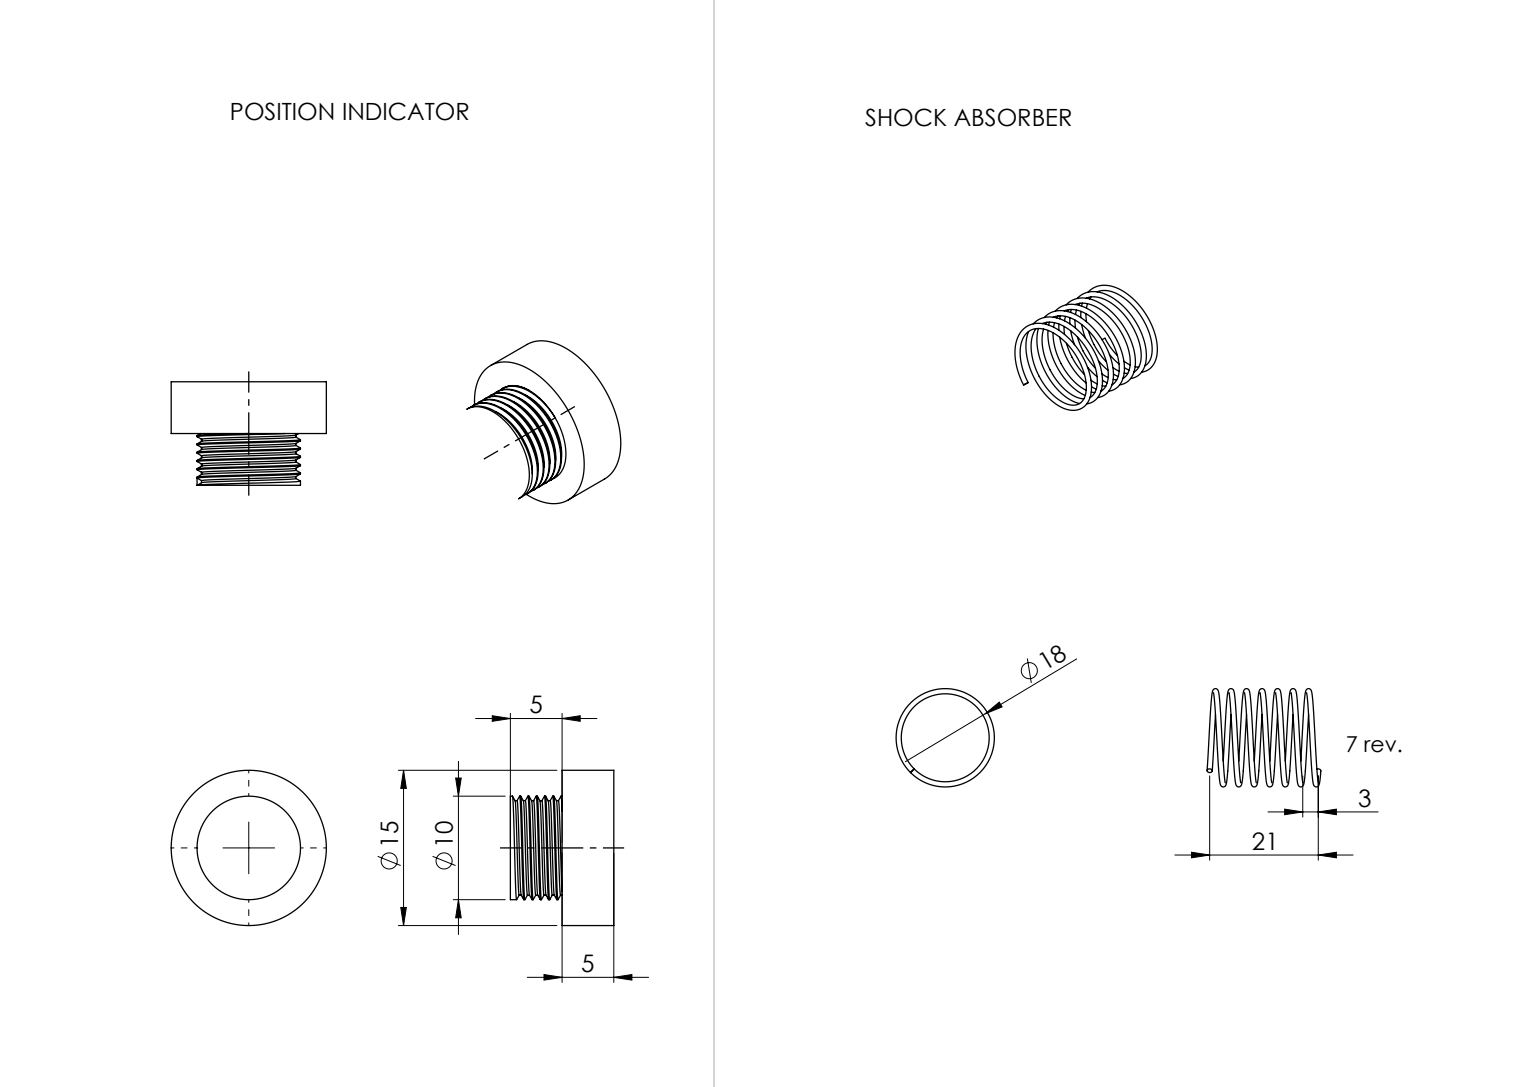
ISO-10303-21;
HEADER;
FILE_DESCRIPTION (('STEP AP214'),
    '1' );
FILE_NAME ('position indicator.step',
    '2026-09-29T11:11:29',
    ( '' ),
    ( '' ),
    'SwSTEP 2.0',
    'SolidWorks 2026',
    '' );
FILE_SCHEMA (( 'AUTOMOTIVE_DESIGN' ));
ENDSEC;

DATA;
#10=FACE_OUTER_BOUND ( 'NONE', #2337, .T. ) ;
#13=CARTESIAN_POINT ( 'NONE',  ( 5.000000000000000000, -47.07106781186545419, -99.34999999781506119 ) ) ;
#14=CARTESIAN_POINT ( 'NONE',  ( -4.566987299999997418, -46.89170807884566727, -96.79999999890753770 ) ) ;
#21=ORIENTED_EDGE ( 'NONE', *, *, #3963, .T. ) ;
#26=CARTESIAN_POINT ( 'NONE',  ( 5.000000000000000000, -47.07106781186545419, -98.54999999781504982 ) ) ;
#27=CARTESIAN_POINT ( 'NONE',  ( 3.535533905932737309, -48.53553390593270933, -96.29999999999999716 ) ) ;
#28=CARTESIAN_POINT ( 'NONE',  ( 9.184850993605145972E-16, -49.99999999999997158, -98.79999999999999716 ) ) ;
#29=ORIENTED_EDGE ( 'NONE', *, *, #4037, .T. ) ;
#33=EDGE_LOOP ( 'NONE', ( #4493, #8102, #3029, #2233, #7688, #6196, #940, #4526, #7806, #8045, #8010, #3978, #7053, #8494, #982 ) ) ;
#34=CARTESIAN_POINT ( 'NONE',  ( 3.229347689422839895, -41.77065231057713390, -98.94999999890752918 ) ) ;
#35=CARTESIAN_POINT ( 'NONE',  ( -4.999999999999997335, -47.07106781186546129, -97.24999999781506688 ) ) ;
#37=CARTESIAN_POINT ( 'NONE',  ( -3.229347689422840784, -41.77065231057713390, -98.54999999890752349 ) ) ;
#38=CARTESIAN_POINT ( 'NONE',  ( 0.000000000000000000, -44.99999999999997158, -100.0000000000000000 ) ) ;
#42=CARTESIAN_POINT ( 'NONE',  ( -3.535533905932735532, -48.53553390593270933, -98.09300000002185982 ) ) ;
#56=CARTESIAN_POINT ( 'NONE',  ( 4.999999999999998224, -42.92893218813449607, -99.24999999781505267 ) ) ;
#60=ADVANCED_FACE ( 'NONE', ( #2297 ), #6169, .T. ) ;
#68=CARTESIAN_POINT ( 'NONE',  ( 4.566987300000000083, -46.89170807884565306, -95.89999999890753202 ) ) ;
#71=VERTEX_POINT ( 'NONE', #7660 ) ;
#75=ORIENTED_EDGE ( 'NONE', *, *, #6394, .T. ) ;
#78=CARTESIAN_POINT ( 'NONE',  ( -1.891708078845683705, -49.56698729999997255, -97.69999999890751496 ) ) ;
#79=CARTESIAN_POINT ( 'NONE',  ( -3.535533905932736864, -41.46446609406723383, -95.79999999781504982 ) ) ;
#81=CARTESIAN_POINT ( 'NONE',  ( -4.566987299999997418, -46.89170807884566727, -99.99999999890754054 ) ) ;
#88=CARTESIAN_POINT ( 'NONE',  ( -4.999999999999998224, -42.92893218813448897, -96.64300000002185698 ) ) ;
#102=FACE_OUTER_BOUND ( 'NONE', #7927, .T. ) ;
#107=CARTESIAN_POINT ( 'NONE',  ( 9.184850993605145972E-16, -49.99999999999997158, -98.79999999999999716 ) ) ;
#114=CARTESIAN_POINT ( 'NONE',  ( 4.566987300000000083, -46.89170807884564596, -95.69999999890752918 ) ) ;
#116=CARTESIAN_POINT ( 'NONE',  ( 0.000000000000000000, -44.99999999999997158, -95.00000000000000000 ) ) ;
#117=CARTESIAN_POINT ( 'NONE',  ( 3.229347689422841228, -48.22934768942280925, -96.74999999890751212 ) ) ;
#119=FACE_OUTER_BOUND ( 'NONE', #8547, .T. ) ;
#126=CARTESIAN_POINT ( 'NONE',  ( 1.891708078845685481, -49.56698729999997255, -96.79999999890752349 ) ) ;
#127=CARTESIAN_POINT ( 'NONE',  ( -3.061616997868382155E-16, -39.99999999999997158, -100.6999999978150555 ) ) ;
#129=CARTESIAN_POINT ( 'NONE',  ( 4.566987299999998307, -44.99999999999997158, -98.04999999890752349 ) ) ;
#130=EDGE_CURVE ( 'NONE', #858, #6099, #1687, .T. ) ;
#132=CARTESIAN_POINT ( 'NONE',  ( -3.061616997868382155E-16, -39.99999999999997158, -98.39300000002185698 ) ) ;
#133=CARTESIAN_POINT ( 'NONE',  ( 4.566987300000000083, -46.89170807884565306, -95.69999999890755760 ) ) ;
#147=CARTESIAN_POINT ( 'NONE',  ( 1.308739421796400793, -40.13013661665839038, -99.99999999999998579 ) ) ;
#149=( NAMED_UNIT ( * ) PLANE_ANGLE_UNIT ( ) SI_UNIT ( $, .RADIAN. ) );
#160=CARTESIAN_POINT ( 'NONE',  ( 3.229347689422841228, -48.22934768942280925, -97.34999999890753486 ) ) ;
#163=CARTESIAN_POINT ( 'NONE',  ( -4.566987299999997418, -46.89170807884566727, -98.59999999890753486 ) ) ;
#172=CARTESIAN_POINT ( 'NONE',  ( -2.071067811865475505, -49.99999999999997158, -98.74999999781503845 ) ) ;
#173=CARTESIAN_POINT ( 'NONE',  ( -3.229347689422839451, -48.22934768942280925, -100.1499999989075178 ) ) ;
#174=CARTESIAN_POINT ( 'NONE',  ( 5.000000000000000000, -47.07106781186545419, -98.54999999781504982 ) ) ;
#175=CARTESIAN_POINT ( 'NONE',  ( 0.000000000000000000, -44.99999999999997158, -100.0000000000000000 ) ) ;
#176=CARTESIAN_POINT ( 'NONE',  ( 4.566987300000000083, -46.89170807884565306, -97.29999999890750928 ) ) ;
#179=CARTESIAN_POINT ( 'NONE',  ( 4.999999999999998224, -42.92893218813448897, -99.34300000002184561 ) ) ;
#180=CARTESIAN_POINT ( 'NONE',  ( -1.891708078845683039, -40.43301269999998482, -96.19999999890752918 ) ) ;
#189=CYLINDRICAL_SURFACE ( 'NONE', #1544, 4.999999999999998224 ) ;
#196=VERTEX_POINT ( 'NONE', #4485 ) ;
#200=EDGE_LOOP ( 'NONE', ( #2778, #541, #7748, #7443, #585 ) ) ;
#201=CARTESIAN_POINT ( 'NONE',  ( -4.566987299999998307, -43.10829192115428299, -96.09999999890753486 ) ) ;
#204=CARTESIAN_POINT ( 'NONE',  ( 4.566987299999998307, -44.99999999999997158, -99.04999999890752349 ) ) ;
#213=CARTESIAN_POINT ( 'NONE',  ( 4.999999999999998224, -44.99999999999997158, -98.60000000000000853 ) ) ;
#214=ADVANCED_FACE ( 'NONE', ( #3002 ), #7128, .T. ) ;
#215=CARTESIAN_POINT ( 'NONE',  ( -3.535533905932735532, -48.53553390593270933, -100.3999999978150441 ) ) ;
#217=CARTESIAN_POINT ( 'NONE',  ( -3.229347689422840784, -41.77065231057713390, -99.34999999890753486 ) ) ;
#221=CARTESIAN_POINT ( 'NONE',  ( 9.184850993605145972E-16, -49.99999999999997158, -99.59300000002184561 ) ) ;
#241=CARTESIAN_POINT ( 'NONE',  ( 4.566987299999998307, -44.99999999999997158, -95.64999999890753202 ) ) ;
#245=CARTESIAN_POINT ( 'NONE',  ( -3.229347689422840784, -41.77065231057713390, -96.34999999890752065 ) ) ;
#246=CARTESIAN_POINT ( 'NONE',  ( 4.999999999999998224, -44.99999999999997158, -95.40000000000000568 ) ) ;
#256=CARTESIAN_POINT ( 'NONE',  ( -3.535533905932736864, -41.46446609406723383, -100.5999999978150470 ) ) ;
#257=EDGE_CURVE ( 'NONE', #6677, #2955, #1349, .T. ) ;
#258=CARTESIAN_POINT ( 'NONE',  ( -4.999999999999998224, -44.99999999999997158, -98.09999999781504698 ) ) ;
#259=CARTESIAN_POINT ( 'NONE',  ( -3.229347689422839451, -48.22934768942280925, -98.34999999890753486 ) ) ;
#264=CARTESIAN_POINT ( 'NONE',  ( 3.535533905932736420, -41.46446609406723383, -95.29999999999999716 ) ) ;
#269=CARTESIAN_POINT ( 'NONE',  ( 4.999999999999998224, -42.92893218813449607, -100.0499999978150640 ) ) ;
#272=CARTESIAN_POINT ( 'NONE',  ( -1.891708078845683039, -40.43301269999998482, -95.59999999890753486 ) ) ;
#281=ADVANCED_FACE ( 'NONE', ( #6423 ), #7751, .T. ) ;
#286=CARTESIAN_POINT ( 'NONE',  ( 1.891708078845682595, -40.43301269999998482, -97.89999999890753202 ) ) ;
#289=CARTESIAN_POINT ( 'NONE',  ( 3.229347689422839895, -41.77065231057713390, -96.54999999890752349 ) ) ;
#291=CARTESIAN_POINT ( 'NONE',  ( -3.229347689422839451, -48.22934768942280925, -98.54999999890752349 ) ) ;
#296=( GEOMETRIC_REPRESENTATION_CONTEXT ( 3 ) GLOBAL_UNCERTAINTY_ASSIGNED_CONTEXT ( ( #1750 ) ) GLOBAL_UNIT_ASSIGNED_CONTEXT ( ( #6287, #2077, #6826 ) ) REPRESENTATION_CONTEXT ( 'NONE', 'WORKASPACE' ) );
#299=DIRECTION ( 'NONE',  ( -1.000000000000000000, 0.000000000000000000, 0.000000000000000000 ) ) ;
#301=CARTESIAN_POINT ( 'NONE',  ( 9.184850993605145972E-16, -49.99999999999997158, -100.2999999978150498 ) ) ;
#304=CARTESIAN_POINT ( 'NONE',  ( -3.229347689422840784, -41.77065231057713390, -100.1499999989075320 ) ) ;
#305=ORIENTED_EDGE ( 'NONE', *, *, #5462, .T. ) ;
#308=CARTESIAN_POINT ( 'NONE',  ( -4.999999999999998224, -45.95670858091268940, -94.97690301168722726 ) ) ;
#309=CARTESIAN_POINT ( 'NONE',  ( -1.891708078845683483, -49.56698729999997255, -95.89999999890753202 ) ) ;
#311=CARTESIAN_POINT ( 'NONE',  ( -2.071067811865475061, -39.99999999999997158, -96.64999999781504414 ) ) ;
#330=CARTESIAN_POINT ( 'NONE',  ( 3.229347689422841228, -48.22934768942280925, -99.94999999890752918 ) ) ;
#332=CARTESIAN_POINT ( 'NONE',  ( 1.891708078845682595, -40.43301269999998482, -95.69999999890751496 ) ) ;
#339=DIRECTION ( 'NONE',  ( -1.000000000000000000, 0.000000000000000000, 0.000000000000000000 ) ) ;
#341=CARTESIAN_POINT ( 'NONE',  ( -2.995331045737738095E-16, -40.10825317499996601, -100.0624999997268958 ) ) ;
#343=CARTESIAN_POINT ( 'NONE',  ( 2.071067811865474173, -39.99999999999997158, -96.85000000000002274 ) ) ;
#347=CARTESIAN_POINT ( 'NONE',  ( 3.535533905932736420, -41.46446609406723383, -97.69999999999998863 ) ) ;
#348=CARTESIAN_POINT ( 'NONE',  ( 4.999999999999998224, -42.92893218813448897, -96.84999999781504698 ) ) ;
#351=ADVANCED_FACE ( 'NONE', ( #3786 ), #5764, .T. ) ;
#354=CARTESIAN_POINT ( 'NONE',  ( -4.999999999999997335, -47.07106781186546129, -97.24999999781505267 ) ) ;
#355=CARTESIAN_POINT ( 'NONE',  ( -4.566987299999998307, -44.99999999999997158, -95.24999999890752633 ) ) ;
#364=ADVANCED_FACE ( 'NONE', ( #6505 ), #5809, .T. ) ;
#365=CARTESIAN_POINT ( 'NONE',  ( -4.566987299999998307, -43.10829192115428299, -99.29999999890752349 ) ) ;
#371=CARTESIAN_POINT ( 'NONE',  ( 4.566987299999998307, -44.99999999999997158, -98.24999999890751212 ) ) ;
#384=CARTESIAN_POINT ( 'NONE',  ( -2.071067811865475505, -49.99999999999996447, -95.64999999999999147 ) ) ;
#388=CARTESIAN_POINT ( 'NONE',  ( -2.071067811865475061, -39.99999999999997158, -96.75000000000001421 ) ) ;
#389=CARTESIAN_POINT ( 'NONE',  ( -4.999999999999998224, -44.99999999999997158, -97.29999999781504982 ) ) ;
#393=CARTESIAN_POINT ( 'NONE',  ( -4.999999999999998224, -42.92893218813449607, -98.25000000000000000 ) ) ;
#398=ORIENTED_EDGE ( 'NONE', *, *, #4779, .F. ) ;
#402=CARTESIAN_POINT ( 'NONE',  ( -4.999999999999998224, -44.99999999999997158, -95.79999999999999716 ) ) ;
#407=CARTESIAN_POINT ( 'NONE',  ( -4.566987299999998307, -44.99999999999997158, -96.24999999890751212 ) ) ;
#409=ORIENTED_EDGE ( 'NONE', *, *, #2203, .F. ) ;
#420=CARTESIAN_POINT ( 'NONE',  ( -2.071067811865475061, -39.99999999999997158, -95.15000000000000568 ) ) ;
#421=ORIENTED_EDGE ( 'NONE', *, *, #5864, .T. ) ;
#423=B_SPLINE_CURVE_WITH_KNOTS ( 'NONE', 3,
 ( #808, #6973, #5609, #147, #3632, #5471 ),
 .UNSPECIFIED., .F., .F.,
 ( 4, 2, 4 ),
 ( 0.1250000000000000000, 0.1875000000000000000, 0.2500000000000000000 ),
 .UNSPECIFIED. ) ;
#426=CARTESIAN_POINT ( 'NONE',  ( -3.061616997868382155E-16, -39.99999999999997158, -99.20000000000000284 ) ) ;
#427=CARTESIAN_POINT ( 'NONE',  ( 2.528021161412670192, -49.35149720828152908, -99.99914980755436034 ) ) ;
#434=CARTESIAN_POINT ( 'NONE',  ( 0.000000000000000000, -44.99999999999997158, -95.00000000000000000 ) ) ;
#442=CARTESIAN_POINT ( 'NONE',  ( 1.891708078845685481, -49.56698729999997255, -98.19999999890752918 ) ) ;
#449=CARTESIAN_POINT ( 'NONE',  ( 1.891708078845682595, -40.43301269999998482, -98.09999999890750644 ) ) ;
#462=CARTESIAN_POINT ( 'NONE',  ( -3.535533905932736864, -41.46446609406723383, -97.50000000000000000 ) ) ;
#468=CARTESIAN_POINT ( 'NONE',  ( -3.061616997868382155E-16, -39.99999999999997158, -97.60000000000000853 ) ) ;
#472=CARTESIAN_POINT ( 'NONE',  ( 4.999999999999998224, -44.99999999999997158, -96.89999999781505835 ) ) ;
#482=CARTESIAN_POINT ( 'NONE',  ( -3.229347689422840784, -41.77065231057713390, -99.34999999890753486 ) ) ;
#486=EDGE_CURVE ( 'NONE', #2955, #4083, #3727, .T. ) ;
#488=CARTESIAN_POINT ( 'NONE',  ( -4.566987299999998307, -44.99999999999997158, -96.04999999890752349 ) ) ;
#502=CARTESIAN_POINT ( 'NONE',  ( 4.999999999999998224, -44.99999999999997158, -97.00000000000000000 ) ) ;
#503=CARTESIAN_POINT ( 'NONE',  ( -3.535533905932736864, -41.46446609406723383, -99.90000000000000568 ) ) ;
#512=CARTESIAN_POINT ( 'NONE',  ( 2.071067811865474173, -39.99999999999997158, -97.64999999999999147 ) ) ;
#514=CARTESIAN_POINT ( 'NONE',  ( -4.961280561519337162, -44.31574741195442613, -99.99919817926395638 ) ) ;
#515=EDGE_CURVE ( 'NONE', #71, #2692, #2215, .T. ) ;
#528=CARTESIAN_POINT ( 'NONE',  ( 4.999999999999998224, -42.92893218813449607, -96.15000000000000568 ) ) ;
#535=CARTESIAN_POINT ( 'NONE',  ( 4.566987299999998307, -44.99999999999997158, -96.44999999890752918 ) ) ;
#541=ORIENTED_EDGE ( 'NONE', *, *, #2221, .F. ) ;
#547=CARTESIAN_POINT ( 'NONE',  ( 3.535533905932736420, -41.46446609406723383, -95.99999999781503845 ) ) ;
#553=CARTESIAN_POINT ( 'NONE',  ( -4.566987299999998307, -43.10829192115428299, -95.49999999890754054 ) ) ;
#554=CARTESIAN_POINT ( 'NONE',  ( 4.999999999999998224, -44.99999999999997158, -97.69999999781505551 ) ) ;
#557=CARTESIAN_POINT ( 'NONE',  ( -3.229347689422839451, -48.22934768942280925, -99.14999999890753202 ) ) ;
#558=CARTESIAN_POINT ( 'NONE',  ( -2.227513643315880643, -40.48620403085396902, -99.99969435636208459 ) ) ;
#561=CARTESIAN_POINT ( 'NONE',  ( 3.535533905932737309, -48.53553390593270933, -97.09300000002185982 ) ) ;
#564=( GEOMETRIC_REPRESENTATION_CONTEXT ( 3 ) GLOBAL_UNCERTAINTY_ASSIGNED_CONTEXT ( ( #7738 ) ) GLOBAL_UNIT_ASSIGNED_CONTEXT ( ( #896, #4163, #2803 ) ) REPRESENTATION_CONTEXT ( 'NONE', 'WORKASPACE' ) );
#578=CARTESIAN_POINT ( 'NONE',  ( 4.566987300000000083, -46.89170807884565306, -99.09999999890752065 ) ) ;
#581=CARTESIAN_POINT ( 'NONE',  ( -4.999999999999998224, -44.99999999999997158, -95.00000000000000000 ) ) ;
#585=ORIENTED_EDGE ( 'NONE', *, *, #701, .F. ) ;
#591=CARTESIAN_POINT ( 'NONE',  ( 4.999999999999998224, -44.99999999999997158, -98.49999999781503845 ) ) ;
#592=CARTESIAN_POINT ( 'NONE',  ( 3.535533905932737309, -48.53553390593270933, -98.59999999781504698 ) ) ;
#593=CARTESIAN_POINT ( 'NONE',  ( 4.999999999999998224, -44.99999999999997158, -95.00000000000000000 ) ) ;
#594=CARTESIAN_POINT ( 'NONE',  ( 3.535533905932736420, -41.46446609406723383, -99.29999999999999716 ) ) ;
#599=CARTESIAN_POINT ( 'NONE',  ( -3.229347689422840784, -41.77065231057713390, -98.74999999890751212 ) ) ;
#600=CARTESIAN_POINT ( 'NONE',  ( -4.999999999999998224, -45.95670858091268940, -95.67690300950226856 ) ) ;
#602=CARTESIAN_POINT ( 'NONE',  ( 4.566987300000000083, -46.89170807884565306, -97.29999999890750928 ) ) ;
#603=CARTESIAN_POINT ( 'NONE',  ( -4.111674810624561971, -47.85923343201969260, -99.99917207927896357 ) ) ;
#607=CARTESIAN_POINT ( 'NONE',  ( -2.071067811865475061, -39.99999999999997158, -97.54300000002184845 ) ) ;
#614=EDGE_LOOP ( 'NONE', ( #6274, #1845, #5331, #7137 ) ) ;
#619=ADVANCED_FACE ( 'NONE', ( #8516 ), #6422, .T. ) ;
#622=CARTESIAN_POINT ( 'NONE',  ( 4.999999999999998224, -44.99999999999997158, -99.29999999781504982 ) ) ;
#624=CARTESIAN_POINT ( 'NONE',  ( -4.566987299999997418, -46.89170807884566727, -99.39999999890751781 ) ) ;
#634=EDGE_LOOP ( 'NONE', ( #2546, #1880, #6420, #7835 ) ) ;
#639=CARTESIAN_POINT ( 'NONE',  ( 1.891708078845682595, -40.43301269999998482, -95.69999999890751496 ) ) ;
#640=CARTESIAN_POINT ( 'NONE',  ( -3.535533905932735532, -48.53553390593270933, -96.50000000000000000 ) ) ;
#641=CARTESIAN_POINT ( 'NONE',  ( -2.071067811865475061, -39.99999999999997158, -99.94999999999998863 ) ) ;
#647=CARTESIAN_POINT ( 'NONE',  ( -1.891708078845683705, -49.56698729999997255, -99.29999999890752349 ) ) ;
#648=CARTESIAN_POINT ( 'NONE',  ( 2.071067811865477282, -49.99999999999996447, -99.54999999999998295 ) ) ;
#650=CARTESIAN_POINT ( 'NONE',  ( 4.566987299999998307, -44.99999999999997158, -98.84999999890753486 ) ) ;
#656=CARTESIAN_POINT ( 'NONE',  ( 4.999999999999998224, -42.92893218813448897, -97.74300000002186550 ) ) ;
#666=ADVANCED_FACE ( 'NONE', ( #7216 ), #4530, .T. ) ;
#672=CARTESIAN_POINT ( 'NONE',  ( 8.389419568037416259E-16, -49.56698729999997255, -100.0499999989075093 ) ) ;
#681=ORIENTED_EDGE ( 'NONE', *, *, #1766, .F. ) ;
#685=CARTESIAN_POINT ( 'NONE',  ( -4.566987299999998307, -44.99999999999997158, -95.44999999890751496 ) ) ;
#687=CARTESIAN_POINT ( 'NONE',  ( 5.000000000000000000, -47.07106781186545419, -99.45000000000000284 ) ) ;
#688=ORIENTED_EDGE ( 'NONE', *, *, #7144, .T. ) ;
#692=ORIENTED_EDGE ( 'NONE', *, *, #3230, .T. ) ;
#693=CARTESIAN_POINT ( 'NONE',  ( 4.566987300000000083, -46.89170807884564596, -97.49999999890752633 ) ) ;
#694=CARTESIAN_POINT ( 'NONE',  ( 4.999999999999998224, -42.92893218813448897, -99.35000000000000853 ) ) ;
#696=CARTESIAN_POINT ( 'NONE',  ( -2.796473189345805913E-16, -40.43301269999997061, -97.04999999890752349 ) ) ;
#700=CARTESIAN_POINT ( 'NONE',  ( -3.061616997868382155E-16, -39.99999999999997158, -95.99300000002185129 ) ) ;
#701=EDGE_CURVE ( 'NONE', #2848, #7832, #7939, .T. ) ;
#707=ORIENTED_EDGE ( 'NONE', *, *, #8464, .T. ) ;
#723=EDGE_CURVE ( 'NONE', #4083, #876, #2542, .T. ) ;
#729=CARTESIAN_POINT ( 'NONE',  ( -4.999999999999998224, -44.99999999999997158, -100.4999999978150385 ) ) ;
#732=( BOUNDED_CURVE ( )  B_SPLINE_CURVE ( 2, ( #402, #3161, #7865, #3114, #1829, #4510, #7198, #528, #4072 ),
 .UNSPECIFIED., .F., .T. ) 
 B_SPLINE_CURVE_WITH_KNOTS ( ( 3, 2, 2, 2, 3 ),
 ( 0.1428571428571428215, 0.1607142857142856984, 0.1785714285714285476, 0.1964285714285714246, 0.2142857142857142738 ),
 .UNSPECIFIED. ) 
 CURVE ( )  GEOMETRIC_REPRESENTATION_ITEM ( )  RATIONAL_B_SPLINE_CURVE ( ( 1.000000000000000222, 0.9238795325112866275, 1.000000000000000000, 0.9238795325112867385, 1.000000000000000000, 0.9238795325112867385, 1.000000000000000000, 0.9238795325112867385, 1.000000000000000000 ) ) 
 REPRESENTATION_ITEM ( '' )  );
#740=CARTESIAN_POINT ( 'NONE',  ( -4.566987299999998307, -44.99999999999997158, -97.84999999890752065 ) ) ;
#741=CARTESIAN_POINT ( 'NONE',  ( 3.535533905932737309, -48.53553390593270933, -99.50000000000000000 ) ) ;
#743=CARTESIAN_POINT ( 'NONE',  ( 3.229347689422841228, -48.22934768942280925, -97.34999999890753486 ) ) ;
#744=SURFACE_SIDE_STYLE ('',( #4672 ) ) ;
#747=CARTESIAN_POINT ( 'NONE',  ( -4.999999999999998224, -42.92893218813448897, -95.04300000002184845 ) ) ;
#753=ORIENTED_EDGE ( 'NONE', *, *, #7226, .F. ) ;
#758=DIRECTION ( 'NONE',  ( 0.000000000000000000, 0.000000000000000000, 1.000000000000000000 ) ) ;
#765=CARTESIAN_POINT ( 'NONE',  ( 4.999999999999998224, -44.99999999999997158, -98.60000000000000853 ) ) ;
#773=CARTESIAN_POINT ( 'NONE',  ( -4.566987299999998307, -44.99999999999997158, -100.0499999989075235 ) ) ;
#775=CARTESIAN_POINT ( 'NONE',  ( -2.071067811865475505, -49.99999999999996447, -98.74999999781503845 ) ) ;
#782=AXIS2_PLACEMENT_3D ( 'NONE', #1939, #5036, #8351 ) ;
#785=CARTESIAN_POINT ( 'NONE',  ( -1.891708078845683705, -49.56698729999997255, -98.49999999890752633 ) ) ;
#786=EDGE_CURVE ( 'NONE', #5319, #2418, #5107, .T. ) ;
#787=CARTESIAN_POINT ( 'NONE',  ( 4.999999999999998224, -42.92893218813448897, -100.0499999978150356 ) ) ;
#789=CARTESIAN_POINT ( 'NONE',  ( 3.229347689422841228, -48.22934768942280925, -98.14999999890753202 ) ) ;
#790=PLANE ( 'NONE',  #5639 ) ;
#793=EDGE_CURVE ( 'NONE', #5525, #6251, #3781, .T. ) ;
#794=CARTESIAN_POINT ( 'NONE',  ( 3.535533905932736420, -41.46446609406723383, -99.29300000002184845 ) ) ;
#797=FACE_OUTER_BOUND ( 'NONE', #8191, .T. ) ;
#799=VERTEX_POINT ( 'NONE', #8543 ) ;
#800=CARTESIAN_POINT ( 'NONE',  ( 4.999999999999998224, -44.99999999999997158, -100.0999999978150470 ) ) ;
#808=CARTESIAN_POINT ( 'NONE',  ( 3.535533969928884801, -41.46446615806338087, -100.0000000000000142 ) ) ;
#811=CARTESIAN_POINT ( 'NONE',  ( 2.071067811865477282, -49.99999999999997158, -98.75000000000001421 ) ) ;
#816=ORIENTED_EDGE ( 'NONE', *, *, #1726, .T. ) ;
#817=CARTESIAN_POINT ( 'NONE',  ( 4.566987299999998307, -43.10829192115428299, -97.19999999890751496 ) ) ;
#821=CARTESIAN_POINT ( 'NONE',  ( 3.229347689422839895, -41.77065231057713390, -97.34999999890752065 ) ) ;
#832=CARTESIAN_POINT ( 'NONE',  ( 3.229347689422841228, -48.22934768942280925, -98.94999999890752918 ) ) ;
#835=CARTESIAN_POINT ( 'NONE',  ( -2.071067811865475061, -39.99999999999997158, -95.15000000000000568 ) ) ;
#836=CARTESIAN_POINT ( 'NONE',  ( 4.566987299999998307, -44.99999999999997158, -96.44999999890752918 ) ) ;
#838=AXIS2_PLACEMENT_3D ( 'NONE', #8397, #5741, #2402 ) ;
#858=VERTEX_POINT ( 'NONE', #591 ) ;
#861=CARTESIAN_POINT ( 'NONE',  ( -2.796473189345805913E-16, -40.43301269999997061, -98.04999999890752349 ) ) ;
#872=CARTESIAN_POINT ( 'NONE',  ( -3.229347689422840784, -41.77065231057713390, -100.3499999989075206 ) ) ;
#873=CARTESIAN_POINT ( 'NONE',  ( -4.999999999999998224, -42.92893218813448897, -98.94999999781504130 ) ) ;
#875=CARTESIAN_POINT ( 'NONE',  ( -1.891708078845683483, -49.56698729999997255, -97.49999999890754054 ) ) ;
#876=VERTEX_POINT ( 'NONE', #8711 ) ;
#879=CARTESIAN_POINT ( 'NONE',  ( -4.999999999999997335, -47.07106781186546129, -98.14300000002184277 ) ) ;
#891=CARTESIAN_POINT ( 'NONE',  ( 0.000000000000000000, -44.99999999999997158, -95.00000000000000000 ) ) ;
#896=( LENGTH_UNIT ( ) NAMED_UNIT ( * ) SI_UNIT ( .MILLI., .METRE. ) );
#905=CARTESIAN_POINT ( 'NONE',  ( -1.891708078845683039, -40.43301269999998482, -100.1999999989075150 ) ) ;
#908=CARTESIAN_POINT ( 'NONE',  ( -3.229347689422840784, -41.77065231057713390, -97.14999999890753202 ) ) ;
#910=CARTESIAN_POINT ( 'NONE',  ( 4.999999999999998224, -44.99999999999997158, -96.09999999781504698 ) ) ;
#916=EDGE_CURVE ( 'NONE', #5583, #5143, #1973, .T. ) ;
#918=CARTESIAN_POINT ( 'NONE',  ( -3.535533905932735532, -48.53553390593270933, -98.79999999781504982 ) ) ;
#920=CARTESIAN_POINT ( 'NONE',  ( -4.999999999999998224, -44.99999999999997158, -98.09999999781504698 ) ) ;
#921=CARTESIAN_POINT ( 'NONE',  ( 9.184850993605145972E-16, -49.99999999999997158, -97.89999999781504414 ) ) ;
#922=CARTESIAN_POINT ( 'NONE',  ( -1.891708078845683483, -49.56698729999997255, -99.89999999890753202 ) ) ;
#927=CARTESIAN_POINT ( 'NONE',  ( -3.535533905932736864, -41.46446609406723383, -99.89300000002185698 ) ) ;
#928=CARTESIAN_POINT ( 'NONE',  ( 4.566987299999998307, -43.10829192115428299, -95.59999999890754907 ) ) ;
#930=CARTESIAN_POINT ( 'NONE',  ( 5.000000000000000000, -47.07106781186545419, -96.94999999781504130 ) ) ;
#940=ORIENTED_EDGE ( 'NONE', *, *, #4323, .F. ) ;
#948=CARTESIAN_POINT ( 'NONE',  ( -2.796473189345805913E-16, -40.43301269999997061, -97.84999999890753486 ) ) ;
#951=CARTESIAN_POINT ( 'NONE',  ( -3.229347689422839451, -48.22934768942280925, -97.74999999890751212 ) ) ;
#953=CARTESIAN_POINT ( 'NONE',  ( 4.566987299999998307, -43.10829192115428299, -96.59999999890753486 ) ) ;
#954=LINE ( 'NONE', #2655, #1137 ) ;
#963=CARTESIAN_POINT ( 'NONE',  ( -4.999999999999998224, -44.99999999999997158, -99.69999999781505551 ) ) ;
#965=CARTESIAN_POINT ( 'NONE',  ( 4.566987299999998307, -44.99999999999997158, -98.84999999890753486 ) ) ;
#970=CARTESIAN_POINT ( 'NONE',  ( -3.535533905932736864, -41.46446609406723383, -98.29300000002184845 ) ) ;
#972=CARTESIAN_POINT ( 'NONE',  ( 4.999999999999998224, -44.99999999999997158, -97.69999999781505551 ) ) ;
#982=ORIENTED_EDGE ( 'NONE', *, *, #7961, .F. ) ;
#987=CARTESIAN_POINT ( 'NONE',  ( -1.891708078845683705, -49.56698729999997255, -99.09999999890753486 ) ) ;
#993=CARTESIAN_POINT ( 'NONE',  ( -4.566987299999998307, -43.10829192115428299, -97.89999999890751781 ) ) ;
#1002=LINE ( 'NONE', #8423, #4723 ) ;
#1003=DIRECTION ( 'NONE',  ( -1.000000000000000000, -6.123233995736960786E-17, 0.000000000000000000 ) ) ;
#1006=CARTESIAN_POINT ( 'NONE',  ( 9.184850993605145972E-16, -49.99999999999997158, -95.60000000000000853 ) ) ;
#1011=CARTESIAN_POINT ( 'NONE',  ( 4.999999999999998224, -44.99999999999997158, -99.40000000000000568 ) ) ;
#1013=CARTESIAN_POINT ( 'NONE',  ( 8.389419568037416259E-16, -49.56698729999997255, -95.84999999890753486 ) ) ;
#1015=CARTESIAN_POINT ( 'NONE',  ( 3.535533905932736420, -41.46446609406723383, -97.59999999781504698 ) ) ;
#1023=CARTESIAN_POINT ( 'NONE',  ( 4.566987300000000083, -46.89170807884564596, -95.89999999890753202 ) ) ;
#1031=EDGE_LOOP ( 'NONE', ( #6594, #5096, #4196, #1185 ) ) ;
#1035=CARTESIAN_POINT ( 'NONE',  ( -4.999999999999998224, -44.99999999999997158, -95.00000000000000000 ) ) ;
#1040=CARTESIAN_POINT ( 'NONE',  ( 3.229347689422839895, -41.77065231057713390, -97.34999999890752065 ) ) ;
#1048=CARTESIAN_POINT ( 'NONE',  ( 0.000000000000000000, -44.99999999999997158, -95.00000000000000000 ) ) ;
#1050=CARTESIAN_POINT ( 'NONE',  ( -3.061616997868382155E-16, -39.99999999999997158, -97.49999999781503845 ) ) ;
#1052=CARTESIAN_POINT ( 'NONE',  ( 2.071067811865474173, -39.99999999999997158, -96.04999999999999716 ) ) ;
#1056=VERTEX_POINT ( 'NONE', #2815 ) ;
#1057=CARTESIAN_POINT ( 'NONE',  ( 9.184850993605145972E-16, -49.99999999999997158, -98.79999999999999716 ) ) ;
#1058=CARTESIAN_POINT ( 'NONE',  ( -3.535533905932735532, -48.53553390593270933, -97.99999999781503845 ) ) ;
#1066=( BOUNDED_SURFACE ( )  B_SPLINE_SURFACE ( 1, 2, ( 
 ( #1706, #4394, #3038, #1615, #4476, #332, #3648, #7162, #3816, #7083, #7743, #2333, #7120, #6326, #5841, #6455, #407, #4305, #2417, #5095, #1661, #2992, #5713, #953, #5137, #7700, #5669, #8371, #6371, #1755, #6497, #7829, #4352, #1082, #7786, #1122, #3079, #5013, #1040, #4437, #5798, #8531, #5053, #8414, #3120, #2378, #3776, #1794, #7032, #993, #3733, #8492, #2456, #449, #6414, #3691, #371, #4969, #5755, #6989, #3167, #7652, #291, #7955, #5927, #5888, #6052, #6621, #4606, #4563, #1333, #1918, #1247, #578, #8619, #3204, #7204, #4034, #8661, #624, #7913, #3945, #1959, #8574, #6712, #2587, #8700, #3903, #7871, #2538, #4646, #6010, #672, #7290, #2627, #8002, #1288, #5257, #5217, #3294, #2498 ),
 ( #5968, #5297, #1166, #3989, #7334, #3333, #6669, #4517, #1879, #3860, #2672, #5178, #5340, #7246, #8043, #2004, #488, #4696, #7381, #1207, #3378, #6580, #1835, #6539, #535, #3245, #2714, #2050, #4739, #5384, #8093, #14, #8681, #1358, #7359, #1313, #696, #6778, #2697, #6645, #6079, #602, #743, #5323, #3316, #5238, #4813, #7447, #4671, #7933, #5365, #4013, #1405, #3402, #8642, #4059, #3448, #4584, #8023, #8068, #1229, #6692, #2608, #5276, #2031, #1984, #37, #7980, #8596, #1942, #2740, #4719, #650, #3359, #8118, #4764, #7268, #5409, #557, #2561, #1900, #3268, #4627, #7311, #6737, #2076, #4101, #7403, #5948, #3926, #1268, #6601, #3968, #6034, #5990, #2654, #773, #8279, #7517, #905, #2241 ) ),
 .UNSPECIFIED., .F., .F., .T. ) 
 B_SPLINE_SURFACE_WITH_KNOTS ( ( 2, 2 ),
 ( 3, 2, 2, 2, 2, 2, 2, 2, 2, 2, 2, 2, 2, 2, 2, 2, 2, 2, 2, 2, 2, 2, 2, 2, 2, 2, 2, 2, 2, 2, 2, 2, 2, 2, 2, 2, 2, 2, 2, 2, 2, 2, 2, 2, 2, 2, 2, 2, 2, 2, 3 ),
 ( 0.000000000000000000, 1.000000000000000000 ),
 ( 0.000000000000000000, 0.01785714285714285615, 0.03571428571428571230, 0.05357142857142856845, 0.07142857142857142461, 0.08928571428571428770, 0.1071428571428571369, 0.1250000000000000000, 0.1428571428571428492, 0.1607142857142857262, 0.1785714285714285754, 0.1964285714285714246, 0.2142857142857142738, 0.2321428571428571508, 0.2500000000000000000, 0.2678571428571428492, 0.2857142857142856984, 0.3035714285714285476, 0.3214285714285714524, 0.3392857142857143016, 0.3571428571428571508, 0.3750000000000000000, 0.3928571428571428492, 0.4107142857142856984, 0.4285714285714285476, 0.4464285714285714524, 0.4642857142857143016, 0.4821428571428571508, 0.5000000000000000000, 0.5178571428571429047, 0.5357142857142856984, 0.5535714285714286031, 0.5714285714285713969, 0.5892857142857143016, 0.6071428571428570953, 0.6250000000000000000, 0.6428571428571429047, 0.6607142857142856984, 0.6785714285714286031, 0.6964285714285713969, 0.7142857142857143016, 0.7321428571428570953, 0.7500000000000000000, 0.7678571428571429047, 0.7857142857142856984, 0.8035714285714286031, 0.8214285714285713969, 0.8392857142857143016, 0.8571428571428570953, 0.8750000000000000000, 0.8928571428571429047 ),
 .UNSPECIFIED. ) 
 GEOMETRIC_REPRESENTATION_ITEM ( )  RATIONAL_B_SPLINE_SURFACE ( (
 ( 1.000000000000000000, 0.9238795325112867385, 1.000000000000000000, 0.9238795325112867385, 1.000000000000000000, 0.9238795325112867385, 1.000000000000000000, 0.9238795325112867385, 1.000000000000000000, 0.9238795325112867385, 1.000000000000000000, 0.9238795325112867385, 1.000000000000000000, 0.9238795325112867385, 1.000000000000000000, 0.9238795325112867385, 1.000000000000000000, 0.9238795325112867385, 1.000000000000000000, 0.9238795325112867385, 1.000000000000000000, 0.9238795325112867385, 1.000000000000000000, 0.9238795325112867385, 1.000000000000000000, 0.9238795325112867385, 1.000000000000000000, 0.9238795325112867385, 1.000000000000000000, 0.9238795325112867385, 1.000000000000000000, 0.9238795325112867385, 1.000000000000000000, 0.9238795325112867385, 1.000000000000000000, 0.9238795325112867385, 1.000000000000000000, 0.9238795325112867385, 1.000000000000000000, 0.9238795325112867385, 1.000000000000000000, 0.9238795325112867385, 1.000000000000000000, 0.9238795325112867385, 1.000000000000000000, 0.9238795325112867385, 1.000000000000000000, 0.9238795325112867385, 1.000000000000000000, 0.9238795325112867385, 1.000000000000000000, 0.9238795325112867385, 1.000000000000000000, 0.9238795325112867385, 1.000000000000000000, 0.9238795325112867385, 1.000000000000000000, 0.9238795325112867385, 1.000000000000000000, 0.9238795325112867385, 1.000000000000000000, 0.9238795325112867385, 1.000000000000000000, 0.9238795325112867385, 1.000000000000000000, 0.9238795325112867385, 1.000000000000000000, 0.9238795325112867385, 1.000000000000000000, 0.9238795325112867385, 1.000000000000000000, 0.9238795325112867385, 1.000000000000000000, 0.9238795325112867385, 1.000000000000000000, 0.9238795325112867385, 1.000000000000000000, 0.9238795325112867385, 1.000000000000000000, 0.9238795325112867385, 1.000000000000000000, 0.9238795325112867385, 1.000000000000000000, 0.9238795325112867385, 1.000000000000000000, 0.9238795325112867385, 1.000000000000000000, 0.9238795325112867385, 1.000000000000000000, 0.9238795325112867385, 1.000000000000000000, 0.9238795325112867385, 1.000000000000000000, 0.9238795325112867385, 1.000000000000000000, 0.9238795325112867385, 1.000000000000000000, 0.9238795325112867385, 1.000000000000000000, 0.9238795325112867385, 1.000000000000000000),
 ( 1.000000000000000000, 0.9238795325112867385, 1.000000000000000000, 0.9238795325112867385, 1.000000000000000000, 0.9238795325112867385, 1.000000000000000000, 0.9238795325112867385, 1.000000000000000000, 0.9238795325112867385, 1.000000000000000000, 0.9238795325112867385, 1.000000000000000000, 0.9238795325112867385, 1.000000000000000000, 0.9238795325112867385, 1.000000000000000000, 0.9238795325112867385, 1.000000000000000000, 0.9238795325112867385, 1.000000000000000000, 0.9238795325112867385, 1.000000000000000000, 0.9238795325112867385, 1.000000000000000000, 0.9238795325112867385, 1.000000000000000000, 0.9238795325112867385, 1.000000000000000000, 0.9238795325112867385, 1.000000000000000000, 0.9238795325112867385, 1.000000000000000000, 0.9238795325112867385, 1.000000000000000000, 0.9238795325112867385, 1.000000000000000000, 0.9238795325112867385, 1.000000000000000000, 0.9238795325112867385, 1.000000000000000000, 0.9238795325112867385, 1.000000000000000000, 0.9238795325112867385, 1.000000000000000000, 0.9238795325112867385, 1.000000000000000000, 0.9238795325112867385, 1.000000000000000000, 0.9238795325112867385, 1.000000000000000000, 0.9238795325112867385, 1.000000000000000000, 0.9238795325112867385, 1.000000000000000000, 0.9238795325112867385, 1.000000000000000000, 0.9238795325112867385, 1.000000000000000000, 0.9238795325112867385, 1.000000000000000000, 0.9238795325112867385, 1.000000000000000000, 0.9238795325112867385, 1.000000000000000000, 0.9238795325112867385, 1.000000000000000000, 0.9238795325112867385, 1.000000000000000000, 0.9238795325112867385, 1.000000000000000000, 0.9238795325112867385, 1.000000000000000000, 0.9238795325112867385, 1.000000000000000000, 0.9238795325112867385, 1.000000000000000000, 0.9238795325112867385, 1.000000000000000000, 0.9238795325112867385, 1.000000000000000000, 0.9238795325112867385, 1.000000000000000000, 0.9238795325112867385, 1.000000000000000000, 0.9238795325112867385, 1.000000000000000000, 0.9238795325112867385, 1.000000000000000000, 0.9238795325112867385, 1.000000000000000000, 0.9238795325112867385, 1.000000000000000000, 0.9238795325112867385, 1.000000000000000000, 0.9238795325112867385, 1.000000000000000000, 0.9238795325112867385, 1.000000000000000000, 0.9238795325112867385, 1.000000000000000000) ) ) 
 REPRESENTATION_ITEM ( '' )  SURFACE ( )  );
#1077=CARTESIAN_POINT ( 'NONE',  ( 8.389419568037416259E-16, -49.56698729999997255, -99.04999999890752349 ) ) ;
#1082=CARTESIAN_POINT ( 'NONE',  ( -4.566987299999998307, -43.10829192115428299, -97.09999999890752065 ) ) ;
#1093=CARTESIAN_POINT ( 'NONE',  ( -4.999999999999998224, -44.99999999999997158, -95.79999999999999716 ) ) ;
#1096=CARTESIAN_POINT ( 'NONE',  ( 4.999999999999998224, -44.99999999999997158, -95.40000000000000568 ) ) ;
#1101=CARTESIAN_POINT ( 'NONE',  ( -3.535533905932736864, -41.46446609406723383, -99.10000000000000853 ) ) ;
#1103=CARTESIAN_POINT ( 'NONE',  ( 4.270369862968768082, -42.33539640546668892, -99.99920780850642643 ) ) ;
#1105=ADVANCED_FACE ( 'NONE', ( #6898 ), #6943, .T. ) ;
#1116=CARTESIAN_POINT ( 'NONE',  ( -1.891708078845683039, -40.43301269999998482, -100.1999999989075292 ) ) ;
#1122=CARTESIAN_POINT ( 'NONE',  ( -1.891708078845683039, -40.43301269999998482, -97.19999999890752918 ) ) ;
#1133=CARTESIAN_POINT ( 'NONE',  ( -4.999999999999998224, -44.99999999999997158, -97.40000000000000568 ) ) ;
#1135=CARTESIAN_POINT ( 'NONE',  ( 2.071067811865477282, -49.99999999999996447, -97.15000000000000568 ) ) ;
#1137=VECTOR ( 'NONE', #1455, 1000.000000000000000 ) ;
#1141=CARTESIAN_POINT ( 'NONE',  ( 4.999999999999998224, -42.92893218813448897, -98.54999999999999716 ) ) ;
#1158=CARTESIAN_POINT ( 'NONE',  ( -4.566987299999997418, -46.89170807884566017, -98.39999999890753202 ) ) ;
#1160=AXIS2_PLACEMENT_3D ( 'NONE', #8260, #1369, #7455 ) ;
#1163=DIRECTION ( 'NONE',  ( -0.000000000000000000, -0.000000000000000000, 1.000000000000000000 ) ) ;
#1166=CARTESIAN_POINT ( 'NONE',  ( -3.229347689422840784, -41.77065231057713390, -95.34999999890753486 ) ) ;
#1180=CARTESIAN_POINT ( 'NONE',  ( -4.999999999999994671, -47.07106781186546840, -96.55000000000001137 ) ) ;
#1181=CARTESIAN_POINT ( 'NONE',  ( -2.071067811865475505, -49.99999999999996447, -98.85000000000002274 ) ) ;
#1185=ORIENTED_EDGE ( 'NONE', *, *, #2970, .F. ) ;
#1186=CARTESIAN_POINT ( 'NONE',  ( -4.999999999999998224, -44.99999999999997158, -97.40000000000000568 ) ) ;
#1207=CARTESIAN_POINT ( 'NONE',  ( -1.891708078845683039, -40.43301269999998482, -96.19999999890752918 ) ) ;
#1220=CARTESIAN_POINT ( 'NONE',  ( -4.999999999999998224, -44.99999999999997158, -99.79999999999999716 ) ) ;
#1221=ORIENTED_EDGE ( 'NONE', *, *, #5114, .F. ) ;
#1227=CARTESIAN_POINT ( 'NONE',  ( 5.000000000000000000, -47.07106781186545419, -96.25000000000000000 ) ) ;
#1229=CARTESIAN_POINT ( 'NONE',  ( 8.389419568037416259E-16, -49.56698729999997255, -98.24999999890752633 ) ) ;
#1233=CARTESIAN_POINT ( 'NONE',  ( 2.071067811865477282, -49.99999999999996447, -96.34300000002185982 ) ) ;
#1247=CARTESIAN_POINT ( 'NONE',  ( 4.566987299999998307, -44.99999999999997158, -99.04999999890752349 ) ) ;
#1250=LINE ( 'NONE', #3948, #2876 ) ;
#1258=CARTESIAN_POINT ( 'NONE',  ( 4.999999999999998224, -42.92893218813448897, -98.44999999781505551 ) ) ;
#1259=CARTESIAN_POINT ( 'NONE',  ( -3.535533905932735532, -48.53553390593270933, -98.10000000000000853 ) ) ;
#1264=CARTESIAN_POINT ( 'NONE',  ( 3.229347689422839895, -41.77065231057713390, -97.34999999890752065 ) ) ;
#1266=CARTESIAN_POINT ( 'NONE',  ( -2.071067811865475061, -39.99999999999997158, -99.94999999999998863 ) ) ;
#1268=CARTESIAN_POINT ( 'NONE',  ( 3.229347689422841228, -48.22934768942280925, -99.74999999890752633 ) ) ;
#1269=CARTESIAN_POINT ( 'NONE',  ( 4.766825771567327230, -43.38335435358479941, -100.0003056439282147 ) ) ;
#1272=CARTESIAN_POINT ( 'NONE',  ( -2.071067811865475505, -49.99999999999996447, -96.44300000002185413 ) ) ;
#1282=AXIS2_PLACEMENT_3D ( 'NONE', #1511, #4204, #6885 ) ;
#1283=CARTESIAN_POINT ( 'NONE',  ( -5.000000000000003553, -42.92893218813449607, -96.64999999999999147 ) ) ;
#1284=DIRECTION ( 'NONE',  ( -0.000000000000000000, -0.000000000000000000, -1.000000000000000000 ) ) ;
#1288=CARTESIAN_POINT ( 'NONE',  ( -4.566987299999998307, -44.99999999999997158, -100.2499999989075121 ) ) ;
#1289=AXIS2_PLACEMENT_3D ( 'NONE', #4498, #7851, #1977 ) ;
#1293=( BOUNDED_CURVE ( )  B_SPLINE_CURVE ( 2, ( #2605, #553, #3265, #272, #8396, #7061, #3021, #2974, #2316, #1023, #4994, #7727, #3715, #7678, #2358, #1641, #6734, #2028, #2121, #7444, #3444, #7356, #4716, #6219, #4098, #7486, #2073, #126, #1402, #3488, #2651, #7400, #4760, #6121, #4143, #4803, #2735, #2825, #1264, #5406, #6775, #693, #8020, #3399, #8064, #78, #4852, #2784, #740, #1355, #2693, #1451, #5449, #8115, #5497, #6689, #8207, #4054, #2166, #8161, #6822, #785, #3965, #6170, #3356, #6642, #599, #6076, #3313, #5987, #34, #8678, #5320, #1980, #4667, #1310, #4010, #647, #6031, #5362, #4184, #6208, #7661, #5586, #6866, #6910, #3003, #4894, #5721, #4227, #2340, #8293, #8250, #6954, #173, #2872, #5544, #8332, #872, #5021, #2209 ),
 .UNSPECIFIED., .F., .T. ) 
 B_SPLINE_CURVE_WITH_KNOTS ( ( 3, 2, 2, 2, 2, 2, 2, 2, 2, 2, 2, 2, 2, 2, 2, 2, 2, 2, 2, 2, 2, 2, 2, 2, 2, 2, 2, 2, 2, 2, 2, 2, 2, 2, 2, 2, 2, 2, 2, 2, 2, 2, 2, 2, 2, 2, 2, 2, 2, 2, 3 ),
 ( 0.000000000000000000, 0.01785714285714285615, 0.03571428571428571230, 0.05357142857142856845, 0.07142857142857142461, 0.08928571428571428770, 0.1071428571428571369, 0.1250000000000000000, 0.1428571428571428492, 0.1607142857142857262, 0.1785714285714285754, 0.1964285714285714246, 0.2142857142857142738, 0.2321428571428571508, 0.2500000000000000000, 0.2678571428571428492, 0.2857142857142856984, 0.3035714285714285476, 0.3214285714285714524, 0.3392857142857143016, 0.3571428571428571508, 0.3750000000000000000, 0.3928571428571428492, 0.4107142857142856984, 0.4285714285714285476, 0.4464285714285714524, 0.4642857142857143016, 0.4821428571428571508, 0.5000000000000000000, 0.5178571428571429047, 0.5357142857142856984, 0.5535714285714286031, 0.5714285714285713969, 0.5892857142857143016, 0.6071428571428570953, 0.6250000000000000000, 0.6428571428571429047, 0.6607142857142856984, 0.6785714285714286031, 0.6964285714285715079, 0.7142857142857143016, 0.7321428571428570953, 0.7500000000000000000, 0.7678571428571429047, 0.7857142857142856984, 0.8035714285714286031, 0.8214285714285713969, 0.8392857142857143016, 0.8571428571428570953, 0.8750000000000000000, 0.8928571428571429047 ),
 .UNSPECIFIED. ) 
 CURVE ( )  GEOMETRIC_REPRESENTATION_ITEM ( )  RATIONAL_B_SPLINE_CURVE ( ( 1.000000000000000000, 0.9238795325112867385, 1.000000000000000000, 0.9238795325112867385, 1.000000000000000000, 0.9238795325112867385, 1.000000000000000000, 0.9238795325112867385, 1.000000000000000000, 0.9238795325112867385, 1.000000000000000000, 0.9238795325112867385, 1.000000000000000000, 0.9238795325112867385, 1.000000000000000000, 0.9238795325112867385, 1.000000000000000000, 0.9238795325112867385, 1.000000000000000000, 0.9238795325112867385, 1.000000000000000000, 0.9238795325112867385, 1.000000000000000000, 0.9238795325112867385, 1.000000000000000000, 0.9238795325112867385, 1.000000000000000000, 0.9238795325112867385, 1.000000000000000000, 0.9238795325112867385, 1.000000000000000000, 0.9238795325112867385, 1.000000000000000000, 0.9238795325112867385, 1.000000000000000000, 0.9238795325112867385, 1.000000000000000000, 0.9238795325112867385, 1.000000000000000000, 0.9238795325112867385, 1.000000000000000000, 0.9238795325112867385, 1.000000000000000000, 0.9238795325112867385, 1.000000000000000000, 0.9238795325112867385, 1.000000000000000000, 0.9238795325112867385, 1.000000000000000000, 0.9238795325112867385, 1.000000000000000000, 0.9238795325112867385, 1.000000000000000000, 0.9238795325112867385, 1.000000000000000000, 0.9238795325112867385, 1.000000000000000000, 0.9238795325112867385, 1.000000000000000000, 0.9238795325112867385, 1.000000000000000000, 0.9238795325112867385, 1.000000000000000000, 0.9238795325112867385, 1.000000000000000000, 0.9238795325112867385, 1.000000000000000000, 0.9238795325112867385, 1.000000000000000000, 0.9238795325112867385, 1.000000000000000000, 0.9238795325112867385, 1.000000000000000000, 0.9238795325112867385, 1.000000000000000000, 0.9238795325112867385, 1.000000000000000000, 0.9238795325112867385, 1.000000000000000000, 0.9238795325112867385, 1.000000000000000000, 0.9238795325112867385, 1.000000000000000000, 0.9238795325112867385, 1.000000000000000000, 0.9238795325112867385, 1.000000000000000000, 0.9238795325112867385, 1.000000000000000000, 0.9238795325112867385, 1.000000000000000000, 0.9238795325112867385, 1.000000000000000000, 0.9238795325112867385, 1.000000000000000000, 0.9238795325112867385, 1.000000000000000000, 0.9238795325112867385, 1.000000000000000000, 0.9238795325112867385, 1.000000000000000000 ) ) 
 REPRESENTATION_ITEM ( '' )  );
#1302=CARTESIAN_POINT ( 'NONE',  ( -3.061616997868382155E-16, -39.99999999999997158, -100.6999999978150555 ) ) ;
#1304=CARTESIAN_POINT ( 'NONE',  ( -4.999999999999997335, -47.07106781186546129, -98.95000000000000284 ) ) ;
#1310=CARTESIAN_POINT ( 'NONE',  ( 1.891708078845685481, -49.56698729999997255, -99.19999999890751496 ) ) ;
#1311=CARTESIAN_POINT ( 'NONE',  ( -3.535533905932735532, -48.53553390593270933, -97.19999999781504130 ) ) ;
#1313=CARTESIAN_POINT ( 'NONE',  ( -1.891708078845683039, -40.43301269999998482, -96.99999999890752633 ) ) ;
#1318=CARTESIAN_POINT ( 'NONE',  ( 4.999999999999998224, -42.92893218813448897, -96.94300000002183992 ) ) ;
#1323=ORIENTED_EDGE ( 'NONE', *, *, #1743, .T. ) ;
#1331=CARTESIAN_POINT ( 'NONE',  ( 2.071067811865474173, -39.99999999999997158, -99.14999999781504414 ) ) ;
#1333=CARTESIAN_POINT ( 'NONE',  ( 3.229347689422839895, -41.77065231057713390, -98.94999999890752918 ) ) ;
#1337=VECTOR ( 'NONE', #6380, 1000.000000000000000 ) ;
#1346=CARTESIAN_POINT ( 'NONE',  ( -3.061616997868382155E-16, -39.99999999999997158, -99.09999999781504698 ) ) ;
#1349=( BOUNDED_CURVE ( )  B_SPLINE_CURVE ( 2, ( #5060, #2339, #8422, #4402, #6463, #3129, #3046, #1847, #7042 ),
 .UNSPECIFIED., .F., .T. ) 
 B_SPLINE_CURVE_WITH_KNOTS ( ( 3, 2, 2, 2, 3 ),
 ( 0.1428571428571428492, 0.1607142857142857262, 0.1785714285714285754, 0.1964285714285714246, 0.2142857142857142738 ),
 .UNSPECIFIED. ) 
 CURVE ( )  GEOMETRIC_REPRESENTATION_ITEM ( )  RATIONAL_B_SPLINE_CURVE ( ( 1.000000000000000000, 0.9238795325112867385, 1.000000000000000000, 0.9238795325112867385, 1.000000000000000000, 0.9238795325112867385, 1.000000000000000000, 0.9238795325112867385, 1.000000000000000000 ) ) 
 REPRESENTATION_ITEM ( '' )  );
#1355=CARTESIAN_POINT ( 'NONE',  ( -4.566987299999998307, -43.10829192115428299, -97.89999999890751781 ) ) ;
#1356=CARTESIAN_POINT ( 'NONE',  ( 2.071067811865474173, -39.99999999999997158, -97.54999999781504982 ) ) ;
#1358=CARTESIAN_POINT ( 'NONE',  ( -4.566987299999998307, -43.10829192115428299, -96.89999999890751781 ) ) ;
#1364=CARTESIAN_POINT ( 'NONE',  ( 3.535533905932736420, -41.46446609406723383, -95.29300000002184845 ) ) ;
#1368=ADVANCED_FACE ( 'NONE', ( #3582 ), #5808, .T. ) ;
#1369=DIRECTION ( 'NONE',  ( 0.000000000000000000, -1.000000000000000000, 0.000000000000000000 ) ) ;
#1393=CARTESIAN_POINT ( 'NONE',  ( -2.796473189345805913E-16, -40.43301269999997061, -95.64999999890753202 ) ) ;
#1397=ORIENTED_EDGE ( 'NONE', *, *, #3272, .F. ) ;
#1402=CARTESIAN_POINT ( 'NONE',  ( 8.389419568037416259E-16, -49.56698729999997255, -96.84999999890752065 ) ) ;
#1403=CARTESIAN_POINT ( 'NONE',  ( 2.071067811865477282, -49.99999999999996447, -96.24999999781505267 ) ) ;
#1405=CARTESIAN_POINT ( 'NONE',  ( -2.796473189345805913E-16, -40.43301269999997061, -97.84999999890753486 ) ) ;
#1409=CARTESIAN_POINT ( 'NONE',  ( -3.535533905932735532, -48.53553390593270933, -97.29300000002184845 ) ) ;
#1415=VERTEX_POINT ( 'NONE', #2066 ) ;
#1424=CARTESIAN_POINT ( 'NONE',  ( -4.999999999999998224, -44.99999999999997158, -98.19999999999998863 ) ) ;
#1436=CARTESIAN_POINT ( 'NONE',  ( -4.566987299999998307, -44.99999999999997158, -95.24999999890752633 ) ) ;
#1440=CARTESIAN_POINT ( 'NONE',  ( 4.999999999999998224, -42.92893218813448897, -99.24999999781506688 ) ) ;
#1451=CARTESIAN_POINT ( 'NONE',  ( -1.891708078845683039, -40.43301269999998482, -97.99999999890752633 ) ) ;
#1452=CARTESIAN_POINT ( 'NONE',  ( -4.999999999999998224, -44.99999999999997158, -98.89999999781504414 ) ) ;
#1453=CARTESIAN_POINT ( 'NONE',  ( -3.535533905932735532, -48.53553390593270933, -97.99999999781503845 ) ) ;
#1454=CARTESIAN_POINT ( 'NONE',  ( -4.566987299999998307, -43.10829192115428299, -100.0999999989075349 ) ) ;
#1455=DIRECTION ( 'NONE',  ( -0.000000000000000000, -0.000000000000000000, -1.000000000000000000 ) ) ;
#1457=CARTESIAN_POINT ( 'NONE',  ( 5.000000000000000000, -47.07106781186545419, -95.45000000000000284 ) ) ;
#1459=CARTESIAN_POINT ( 'NONE',  ( -2.071067811865475061, -39.99999999999997158, -95.84999999781504698 ) ) ;
#1468=CARTESIAN_POINT ( 'NONE',  ( 9.184850993605145972E-16, -49.99999999999997158, -98.00000000000000000 ) ) ;
#1471=CARTESIAN_POINT ( 'NONE',  ( -2.071067811865475505, -49.99999999999997158, -98.85000000000003695 ) ) ;
#1477=CARTESIAN_POINT ( 'NONE',  ( -4.566987299999997418, -46.89170807884566017, -95.99999999890752633 ) ) ;
#1480=CARTESIAN_POINT ( 'NONE',  ( 4.566987299999998307, -44.99999999999997158, -97.44999999890751496 ) ) ;
#1482=CARTESIAN_POINT ( 'NONE',  ( 0.000000000000000000, -44.99999999999997158, -95.00000000000000000 ) ) ;
#1488=CARTESIAN_POINT ( 'NONE',  ( 3.535533905932737309, -48.53553390593270933, -98.59999999781504698 ) ) ;
#1490=CARTESIAN_POINT ( 'NONE',  ( 3.535533905932737309, -48.53553390593270933, -100.1999999978150555 ) ) ;
#1492=CARTESIAN_POINT ( 'NONE',  ( -2.796473189345805913E-16, -40.43301269999997061, -97.04999999890752349 ) ) ;
#1495=CARTESIAN_POINT ( 'NONE',  ( -4.999999999999998224, -44.99999999999997158, -95.79999999999999716 ) ) ;
#1497=CARTESIAN_POINT ( 'NONE',  ( 4.566987299999998307, -44.99999999999997158, -95.64999999890753202 ) ) ;
#1502=CARTESIAN_POINT ( 'NONE',  ( 9.184850993605145972E-16, -49.99999999999997158, -100.2999999978150498 ) ) ;
#1504=LINE ( 'NONE', #581, #8365 ) ;
#1511=CARTESIAN_POINT ( 'NONE',  ( 0.000000000000000000, -44.99999999999997158, -100.0000000000000000 ) ) ;
#1513=ORIENTED_EDGE ( 'NONE', *, *, #3148, .T. ) ;
#1520=CARTESIAN_POINT ( 'NONE',  ( 1.891708078845685481, -49.56698729999997255, -97.39999999890753202 ) ) ;
#1521=CARTESIAN_POINT ( 'NONE',  ( -2.071067811865475061, -39.99999999999997158, -99.95000000000000284 ) ) ;
#1523=CARTESIAN_POINT ( 'NONE',  ( 1.891708078845682595, -40.43301269999998482, -97.29999999890750928 ) ) ;
#1524=DIRECTION ( 'NONE',  ( 0.000000000000000000, 0.000000000000000000, -1.000000000000000000 ) ) ;
#1534=DIRECTION ( 'NONE',  ( 0.000000000000000000, 0.000000000000000000, -1.000000000000000000 ) ) ;
#1535=CARTESIAN_POINT ( 'NONE',  ( 4.566987299999998307, -43.10829192115428299, -99.59999999890756328 ) ) ;
#1540=CARTESIAN_POINT ( 'NONE',  ( -4.999999999999998224, -42.92893218813448897, -99.04300000002184845 ) ) ;
#1542=CARTESIAN_POINT ( 'NONE',  ( -4.566987299999998307, -44.99999999999997158, -96.84999999890753486 ) ) ;
#1544=AXIS2_PLACEMENT_3D ( 'NONE', #891, #5518, #2182 ) ;
#1553=CARTESIAN_POINT ( 'NONE',  ( 3.535533905932737309, -48.53553390593270933, -97.90000000000000568 ) ) ;
#1556=ORIENTED_EDGE ( 'NONE', *, *, #2461, .F. ) ;
#1563=CARTESIAN_POINT ( 'NONE',  ( -3.229347689422839451, -48.22934768942280925, -95.94999999890752918 ) ) ;
#1566=CARTESIAN_POINT ( 'NONE',  ( 8.389419568037416259E-16, -49.56698729999997255, -97.64999999890751781 ) ) ;
#1572=ADVANCED_FACE ( 'NONE', ( #5537 ), #8242, .T. ) ;
#1579=CARTESIAN_POINT ( 'NONE',  ( -3.535533905932736864, -41.46446609406723383, -98.19999999781505551 ) ) ;
#1580=CARTESIAN_POINT ( 'NONE',  ( 3.535533905932736420, -41.46446609406723383, -99.19999999781505551 ) ) ;
#1582=CARTESIAN_POINT ( 'NONE',  ( 1.891708078845685481, -49.56698729999997255, -98.99999999890752633 ) ) ;
#1586=CARTESIAN_POINT ( 'NONE',  ( 5.000000000000000000, -47.07106781186545419, -99.44300000002183992 ) ) ;
#1589=CARTESIAN_POINT ( 'NONE',  ( 2.071067811865474173, -39.99999999999997158, -96.74999999781503845 ) ) ;
#1603=B_SPLINE_CURVE_WITH_KNOTS ( 'NONE', 1,
 ( #4353, #6415 ),
 .UNSPECIFIED., .F., .F.,
 ( 2, 2 ),
 ( 0.000000000000000000, 1.000000000000000000 ),
 .UNSPECIFIED. ) ;
#1610=CARTESIAN_POINT ( 'NONE',  ( -4.566987299999998307, -44.99999999999997158, -97.64999999890753202 ) ) ;
#1613=CARTESIAN_POINT ( 'NONE',  ( -1.891708078845683039, -40.43301269999998482, -97.19999999890752918 ) ) ;
#1615=CARTESIAN_POINT ( 'NONE',  ( -1.891708078845683039, -40.43301269999998482, -95.59999999890753486 ) ) ;
#1624=CARTESIAN_POINT ( 'NONE',  ( -3.535533905932736864, -41.46446609406723383, -98.99999999781503845 ) ) ;
#1626=CARTESIAN_POINT ( 'NONE',  ( -3.229347689422840784, -41.77065231057713390, -97.74999999890752633 ) ) ;
#1630=EDGE_CURVE ( 'NONE', #5319, #6677, #8611, .T. ) ;
#1632=CARTESIAN_POINT ( 'NONE',  ( -4.999999999999997335, -47.07106781186546129, -99.74300000002186550 ) ) ;
#1634=CARTESIAN_POINT ( 'NONE',  ( 9.184850993605145972E-16, -49.99999999999997158, -97.09999999781504698 ) ) ;
#1637=( BOUNDED_CURVE ( )  B_SPLINE_CURVE ( 2, ( #3372, #1283, #7418, #8568, #3983, #6004, #7283, #4733, #7376 ),
 .UNSPECIFIED., .F., .T. ) 
 B_SPLINE_CURVE_WITH_KNOTS ( ( 3, 2, 2, 2, 3 ),
 ( 0.2857142857142856429, 0.3035714285714284921, 0.3214285714285713969, 0.3392857142857142461, 0.3571428571428570953 ),
 .UNSPECIFIED. ) 
 CURVE ( )  GEOMETRIC_REPRESENTATION_ITEM ( )  RATIONAL_B_SPLINE_CURVE ( ( 1.000000000000000222, 0.9238795325112865164, 1.000000000000000000, 0.9238795325112867385, 1.000000000000000000, 0.9238795325112867385, 1.000000000000000000, 0.9238795325112869605, 0.9999999999999997780 ) ) 
 REPRESENTATION_ITEM ( '' )  );
#1639=CARTESIAN_POINT ( 'NONE',  ( -4.999999999999998224, -42.92893218813449607, -100.5499999978150498 ) ) ;
#1641=CARTESIAN_POINT ( 'NONE',  ( -4.566987299999997418, -46.89170807884566017, -96.19999999890751496 ) ) ;
#1655=ADVANCED_FACE ( 'NONE', ( #119 ), #1066, .T. ) ;
#1656=CARTESIAN_POINT ( 'NONE',  ( 1.891708078845682595, -40.43301269999998482, -99.49999999890752633 ) ) ;
#1659=CARTESIAN_POINT ( 'NONE',  ( -4.566987299999998307, -43.10829192115428299, -97.09999999890752065 ) ) ;
#1661=CARTESIAN_POINT ( 'NONE',  ( -2.796473189345805913E-16, -40.43301269999997061, -96.44999999890751496 ) ) ;
#1670=CARTESIAN_POINT ( 'NONE',  ( -3.061616997868382155E-16, -39.99999999999997158, -98.29999999781504982 ) ) ;
#1671=EDGE_CURVE ( 'NONE', #2194, #2812, #4622, .T. ) ;
#1674=CARTESIAN_POINT ( 'NONE',  ( 3.535533905932736420, -41.46446609406723383, -95.29999999999999716 ) ) ;
#1683=CARTESIAN_POINT ( 'NONE',  ( -4.999999999999998224, -44.99999999999997158, -98.09999999781504698 ) ) ;
#1687=( BOUNDED_CURVE ( )  B_SPLINE_CURVE ( 2, ( #3530, #8249, #1488, #4142, #6207, #172, #918, #3613, #5496 ),
 .UNSPECIFIED., .F., .T. ) 
 B_SPLINE_CURVE_WITH_KNOTS ( ( 3, 2, 2, 2, 3 ),
 ( 0.4999999999999999445, 0.5178571428571429047, 0.5357142857142856984, 0.5535714285714286031, 0.5714285714285713969 ),
 .UNSPECIFIED. ) 
 CURVE ( )  GEOMETRIC_REPRESENTATION_ITEM ( )  RATIONAL_B_SPLINE_CURVE ( ( 1.000000000000000222, 0.9238795325112865164, 1.000000000000000000, 0.9238795325112867385, 1.000000000000000000, 0.9238795325112867385, 1.000000000000000000, 0.9238795325112867385, 1.000000000000000000 ) ) 
 REPRESENTATION_ITEM ( '' )  );
#1704=CARTESIAN_POINT ( 'NONE',  ( -1.891708078845683039, -40.43301269999998482, -100.3999999989075178 ) ) ;
#1706=CARTESIAN_POINT ( 'NONE',  ( -4.566987299999998307, -44.99999999999997158, -95.44999999890751496 ) ) ;
#1707=DIRECTION ( 'NONE',  ( 0.000000000000000000, 0.000000000000000000, 1.000000000000000000 ) ) ;
#1709=EDGE_CURVE ( 'NONE', #6150, #799, #7076, .T. ) ;
#1717=CARTESIAN_POINT ( 'NONE',  ( 2.071067811865474173, -39.99999999999997158, -97.54999999781504982 ) ) ;
#1718=STYLED_ITEM ( 'NONE', ( #4912 ), #3705 ) ;
#1720=CARTESIAN_POINT ( 'NONE',  ( 9.184850993605145972E-16, -49.99999999999997158, -98.00000000000000000 ) ) ;
#1726=EDGE_CURVE ( 'NONE', #7832, #2418, #732, .T. ) ;
#1728=CARTESIAN_POINT ( 'NONE',  ( 5.000000000000000000, -47.07106781186545419, -97.04999999999999716 ) ) ;
#1729=CARTESIAN_POINT ( 'NONE',  ( -3.535533905932736864, -41.46446609406723383, -97.39999999781504414 ) ) ;
#1743=EDGE_CURVE ( 'NONE', #2012, #2194, #4557, .T. ) ;
#1749=CARTESIAN_POINT ( 'NONE',  ( -3.229347689422840784, -41.77065231057713390, -100.1499999989075320 ) ) ;
#1750=UNCERTAINTY_MEASURE_WITH_UNIT (LENGTH_MEASURE( 1.000000000000000082E-05 ), #6287, 'distance_accuracy_value', 'NONE');
#1753=DIRECTION ( 'NONE',  ( 1.000000000000000000, 0.000000000000000000, 0.000000000000000000 ) ) ;
#1755=CARTESIAN_POINT ( 'NONE',  ( -1.891708078845683483, -49.56698729999997255, -96.89999999890751781 ) ) ;
#1756=FACE_OUTER_BOUND ( 'NONE', #2107, .T. ) ;
#1759=VECTOR ( 'NONE', #5840, 1000.000000000000000 ) ;
#1763=DIRECTION ( 'NONE',  ( -0.000000000000000000, -0.000000000000000000, -1.000000000000000000 ) ) ;
#1765=CARTESIAN_POINT ( 'NONE',  ( -4.999999999999998224, -42.92893218813449607, -97.34999999781506119 ) ) ;
#1766=EDGE_CURVE ( 'NONE', #5152, #5525, #1637, .T. ) ;
#1768=CARTESIAN_POINT ( 'NONE',  ( -2.071067811865475505, -49.99999999999996447, -96.45000000000000284 ) ) ;
#1771=ORIENTED_EDGE ( 'NONE', *, *, #3148, .F. ) ;
#1773=CARTESIAN_POINT ( 'NONE',  ( -4.999999999999998224, -42.92893218813448897, -99.05000000000001137 ) ) ;
#1774=CARTESIAN_POINT ( 'NONE',  ( -3.535533905932735532, -48.53553390593270933, -96.39999999781505835 ) ) ;
#1789=CARTESIAN_POINT ( 'NONE',  ( -1.891708078845683705, -49.56698729999997255, -98.29999999890752349 ) ) ;
#1792=CARTESIAN_POINT ( 'NONE',  ( -3.229347689422840784, -41.77065231057713390, -100.3499999989075206 ) ) ;
#1794=CARTESIAN_POINT ( 'NONE',  ( -4.566987299999997418, -46.89170807884566727, -97.79999999890752349 ) ) ;
#1808=CARTESIAN_POINT ( 'NONE',  ( -4.999999999999998224, -42.92893218813448897, -95.85000000000002274 ) ) ;
#1813=CARTESIAN_POINT ( 'NONE',  ( 9.184850993605145972E-16, -49.99999999999997158, -98.00000000000000000 ) ) ;
#1814=CARTESIAN_POINT ( 'NONE',  ( -4.680199288021800186, -46.85220489305395830, -100.0000024770419884 ) ) ;
#1817=CLOSED_SHELL ( 'NONE', ( #4289, #8553, #3851, #60, #7347, #1105, #364, #5005, #281, #6132, #4960, #6122, #1572, #351, #4484, #214, #5595, #8637, #619, #7965, #666, #1368, #1655, #4170 ) ) ;
#1825=ORIENTED_EDGE ( 'NONE', *, *, #2748, .T. ) ;
#1829=CARTESIAN_POINT ( 'NONE',  ( -3.061616997868382155E-16, -39.99999999999997158, -96.00000000000000000 ) ) ;
#1833=CARTESIAN_POINT ( 'NONE',  ( -1.891708078845683039, -40.43301269999998482, -99.59999999890754907 ) ) ;
#1835=CARTESIAN_POINT ( 'NONE',  ( 3.229347689422839895, -41.77065231057713390, -96.34999999890753486 ) ) ;
#1845=ORIENTED_EDGE ( 'NONE', *, *, #7701, .T. ) ;
#1847=CARTESIAN_POINT ( 'NONE',  ( 4.999999999999998224, -42.92893218813449607, -96.84999999781504698 ) ) ;
#1850=CARTESIAN_POINT ( 'NONE',  ( -4.999999999999998224, -42.92893218813448897, -97.44999999999998863 ) ) ;
#1855=MECHANICAL_DESIGN_GEOMETRIC_PRESENTATION_REPRESENTATION('',(#1718),#3962);
#1857=CARTESIAN_POINT ( 'NONE',  ( 2.071067811865477282, -49.99999999999996447, -98.75000000000001421 ) ) ;
#1858=CARTESIAN_POINT ( 'NONE',  ( -3.596541285565526991, -41.51505981109065146, -100.0002518188403116 ) ) ;
#1864=CARTESIAN_POINT ( 'NONE',  ( 4.999999999999998224, -44.99999999999997158, -96.09999999781504698 ) ) ;
#1867=EDGE_LOOP ( 'NONE', ( #8128, #692, #1960, #753 ) ) ;
#1870=VECTOR ( 'NONE', #6682, 1000.000000000000000 ) ;
#1879=CARTESIAN_POINT ( 'NONE',  ( 4.566987299999998307, -44.99999999999997158, -95.64999999890753202 ) ) ;
#1880=ORIENTED_EDGE ( 'NONE', *, *, #486, .T. ) ;
#1898=CARTESIAN_POINT ( 'NONE',  ( -4.999999999999998224, -42.92893218813448897, -97.44999999999998863 ) ) ;
#1900=CARTESIAN_POINT ( 'NONE',  ( -4.566987299999998307, -44.99999999999997158, -99.24999999890752633 ) ) ;
#1903=CARTESIAN_POINT ( 'NONE',  ( -4.999999999999998224, -44.99999999999997158, -96.59300000002185982 ) ) ;
#1908=CARTESIAN_POINT ( 'NONE',  ( 2.071067811865477282, -49.99999999999997158, -99.54999999999999716 ) ) ;
#1917=CARTESIAN_POINT ( 'NONE',  ( -7.654042494670954648E-16, -39.99999999999997158, -100.0000000000000000 ) ) ;
#1918=CARTESIAN_POINT ( 'NONE',  ( 4.566987299999998307, -43.10829192115428299, -98.99999999890751212 ) ) ;
#1931=CARTESIAN_POINT ( 'NONE',  ( 5.000000000000000000, -47.07106781186545419, -99.34999999781506119 ) ) ;
#1933=CARTESIAN_POINT ( 'NONE',  ( -4.999999999999997335, -47.07106781186546129, -98.15000000000000568 ) ) ;
#1939=CARTESIAN_POINT ( 'NONE',  ( 0.000000000000000000, -44.99999999999997158, -95.00000000000000000 ) ) ;
#1940=CARTESIAN_POINT ( 'NONE',  ( 2.071067811865477282, -49.99999999999996447, -97.04999999781504982 ) ) ;
#1942=CARTESIAN_POINT ( 'NONE',  ( 1.891708078845682595, -40.43301269999998482, -98.69999999890752918 ) ) ;
#1943=CARTESIAN_POINT ( 'NONE',  ( 4.922040131017533682, -43.95328541805098155, -100.0010338072894172 ) ) ;
#1945=CARTESIAN_POINT ( 'NONE',  ( 3.535533905932737309, -48.53553390593270933, -97.89300000002185698 ) ) ;
#1959=CARTESIAN_POINT ( 'NONE',  ( -3.229347689422840784, -41.77065231057713390, -99.54999999890752349 ) ) ;
#1960=ORIENTED_EDGE ( 'NONE', *, *, #4797, .T. ) ;
#1970=CARTESIAN_POINT ( 'NONE',  ( -4.999999999999997335, -47.07106781186546129, -99.64999999781502993 ) ) ;
#1971=CARTESIAN_POINT ( 'NONE',  ( -3.535533905932736864, -41.46446609406723383, -95.10000000000000853 ) ) ;
#1972=CARTESIAN_POINT ( 'NONE',  ( -3.535533905932736864, -41.46446609406723383, -99.10000000000000853 ) ) ;
#1973=( BOUNDED_CURVE ( )  B_SPLINE_CURVE ( 2, ( #4087, #5225, #2726, #7924, #3345, #5936, #2640, #3304, #3389 ),
 .UNSPECIFIED., .F., .T. ) 
 B_SPLINE_CURVE_WITH_KNOTS ( ( 3, 2, 2, 2, 3 ),
 ( 0.7142857142857143016, 0.7321428571428570953, 0.7500000000000000000, 0.7678571428571429047, 0.7857142857142856984 ),
 .UNSPECIFIED. ) 
 CURVE ( )  GEOMETRIC_REPRESENTATION_ITEM ( )  RATIONAL_B_SPLINE_CURVE ( ( 1.000000000000000000, 0.9238795325112867385, 1.000000000000000000, 0.9238795325112867385, 1.000000000000000000, 0.9238795325112867385, 1.000000000000000000, 0.9238795325112867385, 1.000000000000000000 ) ) 
 REPRESENTATION_ITEM ( '' )  );
#1977=DIRECTION ( 'NONE',  ( -1.000000000000000000, 0.000000000000000000, 0.000000000000000000 ) ) ;
#1979=ORIENTED_EDGE ( 'NONE', *, *, #2086, .F. ) ;
#1980=CARTESIAN_POINT ( 'NONE',  ( 4.566987300000000083, -46.89170807884564596, -99.09999999890752065 ) ) ;
#1981=CARTESIAN_POINT ( 'NONE',  ( 4.999999999999998224, -42.92893218813448897, -96.04999999781504982 ) ) ;
#1984=CARTESIAN_POINT ( 'NONE',  ( -4.566987299999998307, -43.10829192115428299, -98.49999999890752633 ) ) ;
#1989=CARTESIAN_POINT ( 'NONE',  ( -3.061616997868382155E-16, -39.99999999999997158, -95.19300000002185413 ) ) ;
#1998=CARTESIAN_POINT ( 'NONE',  ( 2.071067811865477282, -49.99999999999996447, -97.94300000002185413 ) ) ;
#2000=PLANE ( 'NONE',  #2928 ) ;
#2002=CARTESIAN_POINT ( 'NONE',  ( 0.000000000000000000, -44.99999999999997158, -95.00000000000000000 ) ) ;
#2004=CARTESIAN_POINT ( 'NONE',  ( -4.566987299999997418, -46.89170807884566727, -95.99999999890752633 ) ) ;
#2012=VERTEX_POINT ( 'NONE', #6797 ) ;
#2017=CARTESIAN_POINT ( 'NONE',  ( 4.999999999999998224, -44.99999999999997158, -95.40000000000000568 ) ) ;
#2019=CARTESIAN_POINT ( 'NONE',  ( -4.999999999999997335, -47.07106781186546129, -100.4499999978150413 ) ) ;
#2028=CARTESIAN_POINT ( 'NONE',  ( -4.566987299999998307, -43.10829192115428299, -96.29999999890752349 ) ) ;
#2029=CARTESIAN_POINT ( 'NONE',  ( -4.999999999999998224, -44.99999999999997158, -97.29999999781504982 ) ) ;
#2031=CARTESIAN_POINT ( 'NONE',  ( -4.566987299999998307, -44.99999999999997158, -98.44999999890752918 ) ) ;
#2032=SURFACE_STYLE_USAGE ( .BOTH. , #744 ) ;
#2035=CARTESIAN_POINT ( 'NONE',  ( -3.535533905932735532, -48.53553390593270933, -95.69300000002185413 ) ) ;
#2044=EDGE_CURVE ( 'NONE', #1415, #5592, #3469, .T. ) ;
#2050=CARTESIAN_POINT ( 'NONE',  ( 1.891708078845685481, -49.56698729999997255, -96.59999999890754907 ) ) ;
#2052=ORIENTED_EDGE ( 'NONE', *, *, #723, .T. ) ;
#2054=VECTOR ( 'NONE', #4822, 1000.000000000000000 ) ;
#2064=CARTESIAN_POINT ( 'NONE',  ( -3.535533905932735532, -48.53553390593270933, -98.79999999781504982 ) ) ;
#2066=CARTESIAN_POINT ( 'NONE',  ( 4.999999999999998224, -44.99999999999997158, -95.00000000000000000 ) ) ;
#2073=CARTESIAN_POINT ( 'NONE',  ( 3.229347689422841228, -48.22934768942280925, -96.74999999890751212 ) ) ;
#2074=CARTESIAN_POINT ( 'NONE',  ( 3.535533905932737309, -48.53553390593270933, -97.79999999781504982 ) ) ;
#2076=CARTESIAN_POINT ( 'NONE',  ( 1.891708078845682595, -40.43301269999998482, -99.49999999890754054 ) ) ;
#2077=( NAMED_UNIT ( * ) PLANE_ANGLE_UNIT ( ) SI_UNIT ( $, .RADIAN. ) );
#2082=CARTESIAN_POINT ( 'NONE',  ( 2.071067811865477282, -49.99999999999996447, -95.54300000002184845 ) ) ;
#2086=EDGE_CURVE ( 'NONE', #6099, #5583, #7543, .T. ) ;
#2099=FILL_AREA_STYLE_COLOUR ( '', #5504 ) ;
#2107=EDGE_LOOP ( 'NONE', ( #2052, #1513, #1221, #4024 ) ) ;
#2112=CARTESIAN_POINT ( 'NONE',  ( 2.071067811865474173, -39.99999999999997158, -99.94999999781505551 ) ) ;
#2121=CARTESIAN_POINT ( 'NONE',  ( -3.229347689422840784, -41.77065231057713390, -96.34999999890752065 ) ) ;
#2122=CARTESIAN_POINT ( 'NONE',  ( -3.535533905932735532, -48.53553390593270933, -96.39999999781505835 ) ) ;
#2124=CARTESIAN_POINT ( 'NONE',  ( 3.229347689422839895, -41.77065231057713390, -97.94999999890751496 ) ) ;
#2130=CARTESIAN_POINT ( 'NONE',  ( 4.999999999999998224, -42.92893218813448897, -98.54300000002183424 ) ) ;
#2132=PLANE ( 'NONE',  #1160 ) ;
#2146=EDGE_LOOP ( 'NONE', ( #409, #4929, #6328, #1397 ) ) ;
#2151=CARTESIAN_POINT ( 'NONE',  ( -1.891708078845683705, -49.56698729999997255, -96.69999999890754339 ) ) ;
#2156=CARTESIAN_POINT ( 'NONE',  ( -4.566987299999998307, -43.10829192115428299, -96.29999999890752349 ) ) ;
#2166=CARTESIAN_POINT ( 'NONE',  ( 3.229347689422841228, -48.22934768942280925, -98.34999999890752065 ) ) ;
#2167=CARTESIAN_POINT ( 'NONE',  ( 9.184850993605145972E-16, -49.99999999999997158, -98.69999999781505551 ) ) ;
#2169=CARTESIAN_POINT ( 'NONE',  ( -4.566987299999997418, -46.89170807884566727, -97.59999999890756328 ) ) ;
#2171=CARTESIAN_POINT ( 'NONE',  ( -2.071067811865475505, -49.99999999999996447, -95.64999999999999147 ) ) ;
#2181=DIRECTION ( 'NONE',  ( 1.000000000000000000, 0.000000000000000000, 0.000000000000000000 ) ) ;
#2182=DIRECTION ( 'NONE',  ( -1.000000000000000000, 0.000000000000000000, 0.000000000000000000 ) ) ;
#2186=( NAMED_UNIT ( * ) SI_UNIT ( $, .STERADIAN. ) SOLID_ANGLE_UNIT ( ) );
#2194=VERTEX_POINT ( 'NONE', #355 ) ;
#2195=CARTESIAN_POINT ( 'NONE',  ( 8.389419568037416259E-16, -49.56698729999997255, -97.44999999890751496 ) ) ;
#2198=CARTESIAN_POINT ( 'NONE',  ( -4.566987299999998307, -43.10829192115428299, -98.69999999890752918 ) ) ;
#2203=EDGE_CURVE ( 'NONE', #858, #2422, #3629, .T. ) ;
#2209=CARTESIAN_POINT ( 'NONE',  ( -2.796473189345805913E-16, -40.43301269999997061, -100.4499999989075292 ) ) ;
#2210=CARTESIAN_POINT ( 'NONE',  ( 0.9662756667218486140, -39.99999999999997158, -100.7233279560109622 ) ) ;
#2211=EDGE_CURVE ( 'NONE', #2194, #5592, #8593, .T. ) ;
#2213=CARTESIAN_POINT ( 'NONE',  ( -4.566987299999998307, -44.99999999999997158, -97.64999999890753202 ) ) ;
#2215=( BOUNDED_CURVE ( )  B_SPLINE_CURVE ( 2, ( #7105, #8436, #5781, #5077, #3884, #5911, #8476 ),
 .UNSPECIFIED., .F., .T. ) 
 B_SPLINE_CURVE_WITH_KNOTS ( ( 3, 2, 2, 3 ),
 ( 0.7142857142857143016, 0.7321428571428570953, 0.7500000000000000000, 0.7678571432794624174 ),
 .UNSPECIFIED. ) 
 CURVE ( )  GEOMETRIC_REPRESENTATION_ITEM ( )  RATIONAL_B_SPLINE_CURVE ( ( 1.000000000000000000, 0.9238795325112867385, 1.000000000000000000, 0.9238795325112867385, 1.000000000000000000, 0.9238795325112867385, 1.000000000000000000 ) ) 
 REPRESENTATION_ITEM ( '' )  );
#2217=CARTESIAN_POINT ( 'NONE',  ( -4.999999999999998224, -42.92893218813448897, -95.85000000000002274 ) ) ;
#2218=PRODUCT_DEFINITION_CONTEXT ( 'detailed design', #7404, 'design' ) ;
#2219=CARTESIAN_POINT ( 'NONE',  ( -1.891708078845683483, -49.56698729999997255, -96.69999999890755760 ) ) ;
#2221=EDGE_CURVE ( 'NONE', #5592, #1415, #7114, .T. ) ;
#2222=CARTESIAN_POINT ( 'NONE',  ( -4.999999999999998224, -42.92893218813449607, -95.74999999781503845 ) ) ;
#2224=CARTESIAN_POINT ( 'NONE',  ( -3.535533905932736864, -41.46446609406723383, -100.5999999978150470 ) ) ;
#2233=ORIENTED_EDGE ( 'NONE', *, *, #6027, .F. ) ;
#2241=CARTESIAN_POINT ( 'NONE',  ( -2.796473189345805913E-16, -40.43301269999997061, -100.2499999989075263 ) ) ;
#2244=CARTESIAN_POINT ( 'NONE',  ( 8.389419568037416259E-16, -49.56698729999997255, -96.84999999890752065 ) ) ;
#2255=CARTESIAN_POINT ( 'NONE',  ( -2.071067811865475505, -49.99999999999996447, -98.74999999781503845 ) ) ;
#2257=CARTESIAN_POINT ( 'NONE',  ( -4.566987299999998307, -44.99999999999997158, -98.44999999890752918 ) ) ;
#2260=CARTESIAN_POINT ( 'NONE',  ( 2.071067811865474173, -39.99999999999997158, -98.44300000002185413 ) ) ;
#2261=CARTESIAN_POINT ( 'NONE',  ( 4.566987299999998307, -43.10829192115428299, -96.39999999890753202 ) ) ;
#2262=CARTESIAN_POINT ( 'NONE',  ( -2.071067811865475505, -49.99999999999996447, -96.34999999781506119 ) ) ;
#2273=CARTESIAN_POINT ( 'NONE',  ( -2.071067811865475505, -49.99999999999997158, -98.04999999999999716 ) ) ;
#2274=MECHANICAL_DESIGN_GEOMETRIC_PRESENTATION_REPRESENTATION('',(#5499),#296);
#2282=CARTESIAN_POINT ( 'NONE',  ( 3.229347689422841228, -48.22934768942280925, -96.54999999890752349 ) ) ;
#2285=CARTESIAN_POINT ( 'NONE',  ( 4.566987299999998307, -43.10829192115428299, -98.99999999890751212 ) ) ;
#2288=CARTESIAN_POINT ( 'NONE',  ( 3.535533905932737309, -48.53553390593270933, -96.19999999781504130 ) ) ;
#2297=FACE_OUTER_BOUND ( 'NONE', #8444, .T. ) ;
#2298=CARTESIAN_POINT ( 'NONE',  ( -4.999999999999998224, -44.99999999999997158, -98.09999999781504698 ) ) ;
#2299=CARTESIAN_POINT ( 'NONE',  ( -2.071067811865475505, -49.99999999999996447, -97.94999999781504130 ) ) ;
#2301=CARTESIAN_POINT ( 'NONE',  ( 1.891708078845685481, -49.56698729999997255, -97.39999999890751781 ) ) ;
#2306=CARTESIAN_POINT ( 'NONE',  ( 3.535533905932736420, -41.46446609406723383, -98.49300000002185129 ) ) ;
#2308=CARTESIAN_POINT ( 'NONE',  ( -1.891708078845683039, -40.43301269999998482, -95.39999999890751781 ) ) ;
#2310=CARTESIAN_POINT ( 'NONE',  ( -3.535533905932736864, -41.46446609406723383, -95.79999999781504982 ) ) ;
#2312=CARTESIAN_POINT ( 'NONE',  ( -2.071067811865475505, -49.99999999999997158, -100.3499999978150612 ) ) ;
#2316=CARTESIAN_POINT ( 'NONE',  ( 4.566987299999998307, -44.99999999999997158, -95.84999999890752065 ) ) ;
#2327=EDGE_CURVE ( 'NONE', #2012, #6772, #1293, .T. ) ;
#2328=CARTESIAN_POINT ( 'NONE',  ( -4.566987299999998307, -44.99999999999997158, -99.24999999890752633 ) ) ;
#2331=CARTESIAN_POINT ( 'NONE',  ( 1.891708078845685481, -49.56698729999997255, -97.59999999890754907 ) ) ;
#2332=LINE ( 'NONE', #5668, #8235 ) ;
#2333=CARTESIAN_POINT ( 'NONE',  ( 1.891708078845685481, -49.56698729999997255, -95.99999999890751212 ) ) ;
#2337=EDGE_LOOP ( 'NONE', ( #21, #688 ) ) ;
#2339=CARTESIAN_POINT ( 'NONE',  ( -4.999999999999998224, -42.92893218813449607, -96.54999999781504982 ) ) ;
#2340=CARTESIAN_POINT ( 'NONE',  ( 3.229347689422841228, -48.22934768942280925, -99.94999999890752918 ) ) ;
#2341=CARTESIAN_POINT ( 'NONE',  ( 4.999999999999998224, -42.92893218813448897, -98.44999999781505551 ) ) ;
#2343=CARTESIAN_POINT ( 'NONE',  ( -2.071067811865475061, -39.99999999999997158, -95.95000000000003126 ) ) ;
#2350=CARTESIAN_POINT ( 'NONE',  ( -3.229347689422840784, -41.77065231057713390, -96.14999999890753202 ) ) ;
#2351=CARTESIAN_POINT ( 'NONE',  ( -4.999999999999997335, -47.07106781186546129, -96.44999999781505551 ) ) ;
#2358=CARTESIAN_POINT ( 'NONE',  ( -3.229347689422839451, -48.22934768942280925, -96.14999999890753202 ) ) ;
#2359=CARTESIAN_POINT ( 'NONE',  ( -3.535533905932736864, -41.46446609406723383, -98.29999999999999716 ) ) ;
#2361=EDGE_CURVE ( 'NONE', #6150, #858, #7319, .T. ) ;
#2371=EDGE_CURVE ( 'NONE', #1415, #2848, #1002, .T. ) ;
#2373=CARTESIAN_POINT ( 'NONE',  ( -3.229347689422839451, -48.22934768942280925, -99.94999999890752918 ) ) ;
#2376=CARTESIAN_POINT ( 'NONE',  ( -1.891708078845683483, -49.56698729999997255, -100.0999999989075206 ) ) ;
#2378=CARTESIAN_POINT ( 'NONE',  ( -1.891708078845683483, -49.56698729999997255, -97.69999999890751496 ) ) ;
#2387=CARTESIAN_POINT ( 'NONE',  ( 4.999999999999994671, -42.92893218813449607, -98.44999999781506972 ) ) ;
#2389=CARTESIAN_POINT ( 'NONE',  ( -4.999999999999998224, -44.99999999999997158, -96.49999999781503845 ) ) ;
#2390=CARTESIAN_POINT ( 'NONE',  ( -1.891708078845683039, -40.43301269999998482, -100.1999999989075150 ) ) ;
#2393=EDGE_LOOP ( 'NONE', ( #5113, #4384, #5262, #7550 ) ) ;
#2394=CARTESIAN_POINT ( 'NONE',  ( 3.535533905932737309, -48.53553390593270933, -97.10000000000000853 ) ) ;
#2402=DIRECTION ( 'NONE',  ( -1.000000000000000000, 0.000000000000000000, 0.000000000000000000 ) ) ;
#2415=CARTESIAN_POINT ( 'NONE',  ( 3.229347689422839895, -41.77065231057713390, -99.74999999890751212 ) ) ;
#2417=CARTESIAN_POINT ( 'NONE',  ( -3.229347689422840784, -41.77065231057713390, -96.34999999890752065 ) ) ;
#2418=VERTEX_POINT ( 'NONE', #5677 ) ;
#2422=VERTEX_POINT ( 'NONE', #213 ) ;
#2424=DIRECTION ( 'NONE',  ( -0.000000000000000000, -0.000000000000000000, -1.000000000000000000 ) ) ;
#2429=CARTESIAN_POINT ( 'NONE',  ( 5.000000000000000000, -47.07106781186545419, -96.25000000000000000 ) ) ;
#2434=CARTESIAN_POINT ( 'NONE',  ( 4.999999999999998224, -42.92893218813448897, -96.15000000000000568 ) ) ;
#2435=CARTESIAN_POINT ( 'NONE',  ( -4.999999999999998224, -42.92893218813448897, -98.14999999781504414 ) ) ;
#2451=CARTESIAN_POINT ( 'NONE',  ( 4.566987299999998307, -44.99999999999997158, -98.84999999890753486 ) ) ;
#2455=LINE ( 'NONE', #7651, #1759 ) ;
#2456=CARTESIAN_POINT ( 'NONE',  ( -2.796473189345805913E-16, -40.43301269999997061, -98.04999999890752349 ) ) ;
#2461=EDGE_CURVE ( 'NONE', #7413, #7480, #5633, .T. ) ;
#2466=CARTESIAN_POINT ( 'NONE',  ( -2.071067811865475505, -49.99999999999997158, -97.25000000000000000 ) ) ;
#2468=CARTESIAN_POINT ( 'NONE',  ( -2.796473189345805913E-16, -40.43301269999997061, -100.2499999989075263 ) ) ;
#2474=CARTESIAN_POINT ( 'NONE',  ( 4.999999999999998224, -44.99999999999997158, -96.20000000000000284 ) ) ;
#2475=CARTESIAN_POINT ( 'NONE',  ( 4.921782859443697866, -45.92696902661836589, -99.99920284823379291 ) ) ;
#2491=CARTESIAN_POINT ( 'NONE',  ( -4.566987299999997418, -46.89170807884566017, -99.19999999890751496 ) ) ;
#2495=CARTESIAN_POINT ( 'NONE',  ( -4.566987299999998307, -43.10829192115428299, -100.2999999989075093 ) ) ;
#2498=CARTESIAN_POINT ( 'NONE',  ( -2.796473189345805913E-16, -40.43301269999997061, -100.4499999989075292 ) ) ;
#2511=CARTESIAN_POINT ( 'NONE',  ( 3.535533905932737309, -48.53553390593270933, -97.10000000000000853 ) ) ;
#2513=CARTESIAN_POINT ( 'NONE',  ( 2.071067811865477282, -49.99999999999996447, -96.35000000000000853 ) ) ;
#2518=CARTESIAN_POINT ( 'NONE',  ( -3.535533905932735532, -48.53553390593270933, -98.10000000000000853 ) ) ;
#2519=CARTESIAN_POINT ( 'NONE',  ( 3.812685264810825814, -48.24684725664164375, -100.0006756392447471 ) ) ;
#2524=CARTESIAN_POINT ( 'NONE',  ( 4.999999999999998224, -42.92893218813449607, -97.75000000000001421 ) ) ;
#2536=CARTESIAN_POINT ( 'NONE',  ( 4.566987300000000083, -46.89170807884565306, -99.89999999890751781 ) ) ;
#2538=CARTESIAN_POINT ( 'NONE',  ( 4.566987300000000083, -46.89170807884565306, -99.89999999890751781 ) ) ;
#2542=( BOUNDED_CURVE ( )  B_SPLINE_CURVE ( 2, ( #7712, #1765, #3175, #5063, #1050, #1717, #6465, #7883, #3742 ),
 .UNSPECIFIED., .F., .T. ) 
 B_SPLINE_CURVE_WITH_KNOTS ( ( 3, 2, 2, 2, 3 ),
 ( 0.2857142857142856984, 0.3035714285714285476, 0.3214285714285715079, 0.3392857142857143571, 0.3571428571428572063 ),
 .UNSPECIFIED. ) 
 CURVE ( )  GEOMETRIC_REPRESENTATION_ITEM ( )  RATIONAL_B_SPLINE_CURVE ( ( 1.000000000000000000, 0.9238795325112867385, 1.000000000000000000, 0.9238795325112867385, 1.000000000000000000, 0.9238795325112867385, 1.000000000000000000, 0.9238795325112865164, 1.000000000000000222 ) ) 
 REPRESENTATION_ITEM ( '' )  );
#2546=ORIENTED_EDGE ( 'NONE', *, *, #6773, .F. ) ;
#2550=CARTESIAN_POINT ( 'NONE',  ( 4.999999999999998224, -44.99999999999997158, -95.00000000000000000 ) ) ;
#2552=CARTESIAN_POINT ( 'NONE',  ( 2.071067811865474173, -39.99999999999997158, -98.44999999999998863 ) ) ;
#2554=AXIS2_PLACEMENT_3D ( 'NONE', #7787, #1707, #3692 ) ;
#2558=DIRECTION ( 'NONE',  ( -0.8660254037844382635, 0.000000000000000000, 0.5000000000000005551 ) ) ;
#2559=CARTESIAN_POINT ( 'NONE',  ( -2.071067811865475505, -49.99999999999996447, -96.45000000000000284 ) ) ;
#2561=CARTESIAN_POINT ( 'NONE',  ( -4.566987299999997418, -46.89170807884566727, -99.19999999890751496 ) ) ;
#2562=CARTESIAN_POINT ( 'NONE',  ( 3.425853254208287346, -48.65268606878520075, -99.99975844170711525 ) ) ;
#2571=CARTESIAN_POINT ( 'NONE',  ( -4.999999999999998224, -44.99999999999997158, -97.40000000000000568 ) ) ;
#2582=CARTESIAN_POINT ( 'NONE',  ( 0.000000000000000000, -44.99999999999997158, -105.0000000000000142 ) ) ;
#2587=CARTESIAN_POINT ( 'NONE',  ( 1.891708078845682595, -40.43301269999998482, -99.69999999890752918 ) ) ;
#2598=CARTESIAN_POINT ( 'NONE',  ( 4.999999999999998224, -44.99999999999997158, -100.0999999978150470 ) ) ;
#2605=CARTESIAN_POINT ( 'NONE',  ( -4.566987299999998307, -44.99999999999997158, -95.44999999890751496 ) ) ;
#2606=CARTESIAN_POINT ( 'NONE',  ( -3.061616997868382155E-16, -39.99999999999997158, -100.0000000000000000 ) ) ;
#2608=CARTESIAN_POINT ( 'NONE',  ( -3.229347689422839451, -48.22934768942280925, -98.34999999890753486 ) ) ;
#2609=CARTESIAN_POINT ( 'NONE',  ( -0.8026348516553690748, -49.96717851360725149, -99.99887219979210329 ) ) ;
#2612=CARTESIAN_POINT ( 'NONE',  ( 5.000000000000000000, -47.07106781186545419, -95.44300000002185413 ) ) ;
#2627=CARTESIAN_POINT ( 'NONE',  ( -3.229347689422839451, -48.22934768942280925, -100.1499999989075178 ) ) ;
#2640=CARTESIAN_POINT ( 'NONE',  ( 3.535533905932736420, -41.46446609406723383, -99.29999999999999716 ) ) ;
#2641=CARTESIAN_POINT ( 'NONE',  ( 3.535533905932736420, -41.46446609406723383, -99.19999999781505551 ) ) ;
#2643=CARTESIAN_POINT ( 'NONE',  ( -3.535533905932736864, -41.46446609406723383, -98.29999999999999716 ) ) ;
#2644=ORIENTED_EDGE ( 'NONE', *, *, #916, .F. ) ;
#2651=CARTESIAN_POINT ( 'NONE',  ( -3.229347689422839451, -48.22934768942280925, -96.94999999890751496 ) ) ;
#2652=CARTESIAN_POINT ( 'NONE',  ( -4.999999999999998224, -44.99999999999997158, -95.69999999781504130 ) ) ;
#2654=CARTESIAN_POINT ( 'NONE',  ( -4.566987299999997418, -46.89170807884566727, -99.99999999890754054 ) ) ;
#2655=CARTESIAN_POINT ( 'NONE',  ( 4.999999999999998224, -44.99999999999997158, -95.00000000000000000 ) ) ;
#2658=CARTESIAN_POINT ( 'NONE',  ( -4.999999999999998224, -44.99999999999997158, -95.79300000002184845 ) ) ;
#2668=CARTESIAN_POINT ( 'NONE',  ( -4.999999999999998224, -44.99999999999997158, -95.00000000000000000 ) ) ;
#2672=CARTESIAN_POINT ( 'NONE',  ( 3.229347689422841228, -48.22934768942280925, -95.74999999890752633 ) ) ;
#2685=CARTESIAN_POINT ( 'NONE',  ( 3.535533905932736420, -41.46446609406723383, -98.39999999781504414 ) ) ;
#2686=CARTESIAN_POINT ( 'NONE',  ( 2.071067811865474173, -39.99999999999997158, -95.25000000000000000 ) ) ;
#2692=VERTEX_POINT ( 'NONE', #3254 ) ;
#2693=CARTESIAN_POINT ( 'NONE',  ( -3.229347689422840784, -41.77065231057713390, -97.94999999890751496 ) ) ;
#2694=CARTESIAN_POINT ( 'NONE',  ( 5.000000000000000000, -47.07106781186545419, -96.94999999781504130 ) ) ;
#2695=AXIS2_PLACEMENT_3D ( 'NONE', #5625, #7449, #8119 ) ;
#2697=CARTESIAN_POINT ( 'NONE',  ( 3.229347689422839895, -41.77065231057713390, -97.14999999890753202 ) ) ;
#2700=CARTESIAN_POINT ( 'NONE',  ( 9.184850993605145972E-16, -49.99999999999997158, -97.99300000002185129 ) ) ;
#2706=CARTESIAN_POINT ( 'NONE',  ( -3.535533905932735532, -48.53553390593270933, -99.70000000000000284 ) ) ;
#2713=CARTESIAN_POINT ( 'NONE',  ( 9.184850993605145972E-16, -49.99999999999997158, -99.49999999781503845 ) ) ;
#2714=CARTESIAN_POINT ( 'NONE',  ( 3.229347689422841228, -48.22934768942280925, -96.54999999890752349 ) ) ;
#2726=CARTESIAN_POINT ( 'NONE',  ( -3.535533905932736864, -41.46446609406723383, -99.10000000000000853 ) ) ;
#2727=CARTESIAN_POINT ( 'NONE',  ( -2.071067811865475061, -39.99999999999997158, -99.04999999781504982 ) ) ;
#2728=CARTESIAN_POINT ( 'NONE',  ( 2.071067811865477282, -49.99999999999997158, -96.35000000000000853 ) ) ;
#2729=CARTESIAN_POINT ( 'NONE',  ( -2.071067811865475505, -49.99999999999996447, -99.64999999999999147 ) ) ;
#2735=CARTESIAN_POINT ( 'NONE',  ( -2.796473189345805913E-16, -40.43301269999997061, -97.24999999890751212 ) ) ;
#2738=CARTESIAN_POINT ( 'NONE',  ( 3.535533905932736420, -41.46446609406723383, -97.59999999781504698 ) ) ;
#2740=CARTESIAN_POINT ( 'NONE',  ( 3.229347689422839895, -41.77065231057713390, -98.74999999890752633 ) ) ;
#2742=DIRECTION ( 'NONE',  ( 0.000000000000000000, 0.000000000000000000, -1.000000000000000000 ) ) ;
#2746=CARTESIAN_POINT ( 'NONE',  ( -4.999999999999997335, -47.07106781186546129, -95.74300000002187971 ) ) ;
#2748=EDGE_CURVE ( 'NONE', #7480, #2812, #5066, .T. ) ;
#2759=FACE_OUTER_BOUND ( 'NONE', #3211, .T. ) ;
#2775=CARTESIAN_POINT ( 'NONE',  ( 3.229347689422841228, -48.22934768942280925, -95.94999999890751496 ) ) ;
#2778=ORIENTED_EDGE ( 'NONE', *, *, #2371, .F. ) ;
#2784=CARTESIAN_POINT ( 'NONE',  ( -4.566987299999997418, -46.89170807884566017, -97.79999999890752349 ) ) ;
#2785=CARTESIAN_POINT ( 'NONE',  ( -4.999999999999997335, -47.07106781186546129, -99.75000000000001421 ) ) ;
#2788=CARTESIAN_POINT ( 'NONE',  ( -3.229347689422840784, -41.77065231057713390, -96.94999999890751496 ) ) ;
#2792=CARTESIAN_POINT ( 'NONE',  ( -2.071067811865475505, -49.99999999999996447, -95.64300000002185698 ) ) ;
#2803=( NAMED_UNIT ( * ) SI_UNIT ( $, .STERADIAN. ) SOLID_ANGLE_UNIT ( ) );
#2805=CARTESIAN_POINT ( 'NONE',  ( 5.000000000000000000, -47.07106781186545419, -98.65000000000000568 ) ) ;
#2812=VERTEX_POINT ( 'NONE', #4791 ) ;
#2813=CARTESIAN_POINT ( 'NONE',  ( 1.891708078845685481, -49.56698729999997255, -95.79999999890752349 ) ) ;
#2815=CARTESIAN_POINT ( 'NONE',  ( -7.499999999999999112, -44.99999999999997158, -105.0000000000000142 ) ) ;
#2816=CARTESIAN_POINT ( 'NONE',  ( -4.566987299999998307, -44.99999999999997158, -96.24999999890751212 ) ) ;
#2818=CARTESIAN_POINT ( 'NONE',  ( -4.999999999999997335, -47.07106781186546129, -96.44999999781504130 ) ) ;
#2825=CARTESIAN_POINT ( 'NONE',  ( 1.891708078845682595, -40.43301269999998482, -97.29999999890752349 ) ) ;
#2826=CARTESIAN_POINT ( 'NONE',  ( 5.000000000000000000, -47.07106781186545419, -100.1499999978150441 ) ) ;
#2828=CARTESIAN_POINT ( 'NONE',  ( -1.891708078845683039, -40.43301269999998482, -97.79999999890752349 ) ) ;
#2831=CARTESIAN_POINT ( 'NONE',  ( 0.9662756667218486140, -39.99999999999997158, -100.0163279582177722 ) ) ;
#2833=CARTESIAN_POINT ( 'NONE',  ( -2.796473189345805913E-16, -40.43301269999997061, -96.24999999890752633 ) ) ;
#2848=VERTEX_POINT ( 'NONE', #2017 ) ;
#2856=CARTESIAN_POINT ( 'NONE',  ( -1.891708078845683705, -49.56698729999997255, -97.49999999890752633 ) ) ;
#2858=VECTOR ( 'NONE', #5679, 1000.000000000000000 ) ;
#2860=CARTESIAN_POINT ( 'NONE',  ( -2.796473189345805913E-16, -40.43301269999997061, -97.24999999890751212 ) ) ;
#2872=CARTESIAN_POINT ( 'NONE',  ( -4.566987299999997418, -46.89170807884566017, -100.1999999989075292 ) ) ;
#2873=CARTESIAN_POINT ( 'NONE',  ( -4.999999999999997335, -47.07106781186546129, -99.64999999781502993 ) ) ;
#2875=CARTESIAN_POINT ( 'NONE',  ( 8.389419568037416259E-16, -49.56698729999997255, -99.04999999890752349 ) ) ;
#2876=VECTOR ( 'NONE', #6624, 1000.000000000000000 ) ;
#2878=CARTESIAN_POINT ( 'NONE',  ( -3.061616997868382155E-16, -39.99999999999997158, -99.99300000002185129 ) ) ;
#2883=( BOUNDED_CURVE ( )  B_SPLINE_CURVE ( 2, ( #7146, #393, #2359, #3101, #7679, #5037, #3757, #6971, #6442 ),
 .UNSPECIFIED., .F., .T. ) 
 B_SPLINE_CURVE_WITH_KNOTS ( ( 3, 2, 2, 2, 3 ),
 ( 0.5714285714285713969, 0.5892857142857143016, 0.6071428571428570953, 0.6250000000000000000, 0.6428571428571429047 ),
 .UNSPECIFIED. ) 
 CURVE ( )  GEOMETRIC_REPRESENTATION_ITEM ( )  RATIONAL_B_SPLINE_CURVE ( ( 1.000000000000000000, 0.9238795325112867385, 1.000000000000000000, 0.9238795325112867385, 1.000000000000000000, 0.9238795325112867385, 1.000000000000000000, 0.9238795325112867385, 1.000000000000000000 ) ) 
 REPRESENTATION_ITEM ( '' )  );
#2894=B_SPLINE_CURVE_WITH_KNOTS ( 'NONE', 1,
 ( #6451, #5663 ),
 .UNSPECIFIED., .F., .F.,
 ( 2, 2 ),
 ( 0.000000000000000000, 1.000000000000000000 ),
 .UNSPECIFIED. ) ;
#2895=SHAPE_REPRESENTATION_RELATIONSHIP ( 'NONE' , 'NONE' ,  #6471, #3705 ) ;
#2904=CARTESIAN_POINT ( 'NONE',  ( 1.891708078845682595, -40.43301269999998482, -96.29999999890752349 ) ) ;
#2906=CARTESIAN_POINT ( 'NONE',  ( 4.566987300000000083, -46.89170807884565306, -99.09999999890752065 ) ) ;
#2919=CARTESIAN_POINT ( 'NONE',  ( 8.389419568037416259E-16, -49.56698729999997255, -98.24999999890752633 ) ) ;
#2921=ORIENTED_EDGE ( 'NONE', *, *, #2211, .T. ) ;
#2923=CARTESIAN_POINT ( 'NONE',  ( 4.999999999999998224, -44.99999999999997158, -99.39300000002185698 ) ) ;
#2927=AXIS2_PLACEMENT_3D ( 'NONE', #116, #6283, #8195 ) ;
#2928=AXIS2_PLACEMENT_3D ( 'NONE', #2582, #4073, #8657 ) ;
#2939=ORIENTED_EDGE ( 'NONE', *, *, #2461, .T. ) ;
#2943=CARTESIAN_POINT ( 'NONE',  ( 4.566987299999998307, -43.10829192115428299, -95.59999999890754907 ) ) ;
#2946=CARTESIAN_POINT ( 'NONE',  ( 1.891708078845685481, -49.56698729999997255, -98.39999999890753202 ) ) ;
#2948=CARTESIAN_POINT ( 'NONE',  ( 9.184850993605145972E-16, -49.99999999999997158, -96.29999999781504982 ) ) ;
#2955=VERTEX_POINT ( 'NONE', #7648 ) ;
#2960=CARTESIAN_POINT ( 'NONE',  ( -3.535533905932735532, -48.53553390593270933, -98.79999999781504982 ) ) ;
#2962=CARTESIAN_POINT ( 'NONE',  ( -3.229347689422839451, -48.22934768942280925, -99.14999999890753202 ) ) ;
#2966=CARTESIAN_POINT ( 'NONE',  ( -4.999999999999998224, -42.92893218813448897, -98.24300000002185129 ) ) ;
#2968=CARTESIAN_POINT ( 'NONE',  ( -4.999999999999998224, -44.99999999999997158, -96.49999999781503845 ) ) ;
#2970=EDGE_CURVE ( 'NONE', #7654, #7480, #7041, .T. ) ;
#2973=PRODUCT_DEFINITION_SHAPE ( 'NONE', 'NONE',  #5874 ) ;
#2974=CARTESIAN_POINT ( 'NONE',  ( 4.566987299999998307, -43.10829192115428299, -95.79999999890752349 ) ) ;
#2978=AXIS2_PLACEMENT_3D ( 'NONE', #3039, #6372, #5842 ) ;
#2988=CARTESIAN_POINT ( 'NONE',  ( 4.566987299999998307, -43.10829192115428299, -97.99999999890752633 ) ) ;
#2990=CARTESIAN_POINT ( 'NONE',  ( 3.229347689422841228, -48.22934768942280925, -98.34999999890752065 ) ) ;
#2992=CARTESIAN_POINT ( 'NONE',  ( 1.891708078845682595, -40.43301269999998482, -96.49999999890752633 ) ) ;
#3002=FACE_OUTER_BOUND ( 'NONE', #3862, .T. ) ;
#3003=CARTESIAN_POINT ( 'NONE',  ( 3.229347689422839895, -41.77065231057713390, -99.74999999890751212 ) ) ;
#3004=CARTESIAN_POINT ( 'NONE',  ( 4.999999999999998224, -42.92893218813448897, -99.24999999781506688 ) ) ;
#3005=CARTESIAN_POINT ( 'NONE',  ( -4.999999999999998224, -44.99999999999997158, -95.00000000000000000 ) ) ;
#3006=CARTESIAN_POINT ( 'NONE',  ( -4.999999999999998224, -44.99999999999997158, -95.79999999999999716 ) ) ;
#3010=CARTESIAN_POINT ( 'NONE',  ( 2.071067811865474173, -39.99999999999997158, -95.25000000000000000 ) ) ;
#3013=CARTESIAN_POINT ( 'NONE',  ( 3.535533905932736420, -41.46446609406723383, -96.79999999781504982 ) ) ;
#3021=CARTESIAN_POINT ( 'NONE',  ( 3.229347689422839895, -41.77065231057713390, -95.74999999890751212 ) ) ;
#3029=ORIENTED_EDGE ( 'NONE', *, *, #8716, .T. ) ;
#3033=CARTESIAN_POINT ( 'NONE',  ( -3.229347689422839451, -48.22934768942280925, -98.34999999890753486 ) ) ;
#3036=CARTESIAN_POINT ( 'NONE',  ( -2.796473189345805913E-16, -40.43301269999997061, -100.4499999989075292 ) ) ;
#3038=CARTESIAN_POINT ( 'NONE',  ( -3.229347689422840784, -41.77065231057713390, -95.54999999890752349 ) ) ;
#3039=CARTESIAN_POINT ( 'NONE',  ( 0.000000000000000000, -44.99999999999997158, -95.00000000000000000 ) ) ;
#3040=ORIENTED_EDGE ( 'NONE', *, *, #6027, .T. ) ;
#3046=CARTESIAN_POINT ( 'NONE',  ( 3.535533905932736420, -41.46446609406723383, -96.79999999781504982 ) ) ;
#3051=CARTESIAN_POINT ( 'NONE',  ( -3.535533905932735532, -48.53553390593270933, -97.29999999999999716 ) ) ;
#3055=CARTESIAN_POINT ( 'NONE',  ( 4.999999999999998224, -42.92893218813448897, -97.75000000000001421 ) ) ;
#3056=CARTESIAN_POINT ( 'NONE',  ( 2.071067811865477282, -49.99999999999996447, -97.04999999781504982 ) ) ;
#3066=DIRECTION ( 'NONE',  ( -0.000000000000000000, -0.000000000000000000, -1.000000000000000000 ) ) ;
#3074=CARTESIAN_POINT ( 'NONE',  ( -2.796473189345805913E-16, -40.43301269999997061, -99.44999999890752918 ) ) ;
#3079=CARTESIAN_POINT ( 'NONE',  ( -2.796473189345805913E-16, -40.43301269999997061, -97.24999999890751212 ) ) ;
#3086=DIRECTION ( 'NONE',  ( -0.000000000000000000, -0.000000000000000000, 1.000000000000000000 ) ) ;
#3090=CARTESIAN_POINT ( 'NONE',  ( -3.061616997868382155E-16, -39.99999999999997158, -96.00000000000000000 ) ) ;
#3091=ORIENTED_EDGE ( 'NONE', *, *, #6940, .F. ) ;
#3094=CARTESIAN_POINT ( 'NONE',  ( -2.071067811865475505, -49.99999999999996447, -98.85000000000002274 ) ) ;
#3101=CARTESIAN_POINT ( 'NONE',  ( -2.071067811865475061, -39.99999999999997158, -98.35000000000000853 ) ) ;
#3105=EDGE_CURVE ( 'NONE', #6677, #5152, #1504, .T. ) ;
#3112=( BOUNDED_CURVE ( )  B_SPLINE_CURVE ( 2, ( #765, #2805, #6755, #811, #107, #1471, #4165, #5301, #8004 ),
 .UNSPECIFIED., .F., .F. ) 
 B_SPLINE_CURVE_WITH_KNOTS ( ( 3, 2, 2, 2, 3 ),
 ( 0.6428571428571429047, 0.6607142857142856984, 0.6785714285714286031, 0.6964285714285713969, 0.7142857142857143016 ),
 .UNSPECIFIED. ) 
 CURVE ( )  GEOMETRIC_REPRESENTATION_ITEM ( )  RATIONAL_B_SPLINE_CURVE ( ( 1.000000000000000000, 0.9238795325112867385, 1.000000000000000000, 0.9238795325112867385, 1.000000000000000000, 0.9238795325112867385, 1.000000000000000000, 0.9238795325112867385, 1.000000000000000000 ) ) 
 REPRESENTATION_ITEM ( '' )  );
#3113=EDGE_CURVE ( 'NONE', #196, #7832, #7874, .T. ) ;
#3114=CARTESIAN_POINT ( 'NONE',  ( -2.071067811865475061, -39.99999999999997158, -95.95000000000001705 ) ) ;
#3118=CARTESIAN_POINT ( 'NONE',  ( 4.566987299999998307, -44.99999999999997158, -99.84999999890752065 ) ) ;
#3120=CARTESIAN_POINT ( 'NONE',  ( 8.389419568037416259E-16, -49.56698729999997255, -97.64999999890751781 ) ) ;
#3129=CARTESIAN_POINT ( 'NONE',  ( 2.071067811865474173, -39.99999999999997158, -96.74999999781503845 ) ) ;
#3132=CARTESIAN_POINT ( 'NONE',  ( 5.000000000000004441, -47.07106781186543998, -97.04999999999999716 ) ) ;
#3135=CARTESIAN_POINT ( 'NONE',  ( 5.000000000000000000, -47.07106781186545419, -95.45000000000000284 ) ) ;
#3141=CARTESIAN_POINT ( 'NONE',  ( 2.071067811865474173, -39.99999999999997158, -99.25000000000000000 ) ) ;
#3143=CARTESIAN_POINT ( 'NONE',  ( 3.991994717416610161, -48.02431555730691315, -100.0008018208966831 ) ) ;
#3145=CYLINDRICAL_SURFACE ( 'NONE', #1289, 4.999999999999998224 ) ;
#3148=EDGE_CURVE ( 'NONE', #876, #4620, #4479, .T. ) ;
#3161=CARTESIAN_POINT ( 'NONE',  ( -5.000000000000000888, -42.92893218813449607, -95.85000000000000853 ) ) ;
#3166=DIRECTION ( 'NONE',  ( 0.000000000000000000, 0.000000000000000000, -1.000000000000000000 ) ) ;
#3167=CARTESIAN_POINT ( 'NONE',  ( 8.389419568037416259E-16, -49.56698729999997255, -98.44999999890752918 ) ) ;
#3175=CARTESIAN_POINT ( 'NONE',  ( -3.535533905932736864, -41.46446609406723383, -97.39999999781504414 ) ) ;
#3177=CARTESIAN_POINT ( 'NONE',  ( -3.061616997868382155E-16, -39.99999999999997158, -97.60000000000000853 ) ) ;
#3182=CARTESIAN_POINT ( 'NONE',  ( 5.000000000000000000, -47.07106781186545419, -97.85000000000002274 ) ) ;
#3183=CARTESIAN_POINT ( 'NONE',  ( -4.581831634694143673, -42.91680744104596101, -100.0003077338198381 ) ) ;
#3197=CARTESIAN_POINT ( 'NONE',  ( 4.566987299999998307, -43.10829192115428299, -99.59999999890754907 ) ) ;
#3202=CARTESIAN_POINT ( 'NONE',  ( -4.999999999999998224, -44.99999999999997158, -98.89999999781504414 ) ) ;
#3204=CARTESIAN_POINT ( 'NONE',  ( 1.891708078845685481, -49.56698729999997255, -99.19999999890751496 ) ) ;
#3211=EDGE_LOOP ( 'NONE', ( #6063, #3558 ) ) ;
#3214=CARTESIAN_POINT ( 'NONE',  ( 2.071067811865477282, -49.99999999999997158, -97.15000000000000568 ) ) ;
#3216=CARTESIAN_POINT ( 'NONE',  ( 9.184850993605145972E-16, -49.99999999999997158, -96.40000000000000568 ) ) ;
#3222=CARTESIAN_POINT ( 'NONE',  ( 4.999999999999998224, -44.99999999999997158, -95.00000000000000000 ) ) ;
#3224=CARTESIAN_POINT ( 'NONE',  ( 2.071067811865477282, -49.99999999999996447, -97.15000000000000568 ) ) ;
#3226=CARTESIAN_POINT ( 'NONE',  ( -7.654042494670954648E-16, -39.99999999999997158, -100.0000000000000000 ) ) ;
#3230=EDGE_CURVE ( 'NONE', #1056, #6586, #1250, .T. ) ;
#3238=CIRCLE ( 'NONE', #838, 7.499999999999999112 ) ;
#3245=CARTESIAN_POINT ( 'NONE',  ( 4.566987300000000083, -46.89170807884565306, -96.49999999890752633 ) ) ;
#3254=CARTESIAN_POINT ( 'NONE',  ( 3.535533969928884801, -41.46446615806338087, -100.0000000000000142 ) ) ;
#3256=CARTESIAN_POINT ( 'NONE',  ( 4.999999999999998224, -42.92893218813448897, -96.04999999781504982 ) ) ;
#3258=CARTESIAN_POINT ( 'NONE',  ( -2.071067811865475061, -39.99999999999997158, -99.14999999999999147 ) ) ;
#3265=CARTESIAN_POINT ( 'NONE',  ( -3.229347689422840784, -41.77065231057713390, -95.54999999890752349 ) ) ;
#3266=CARTESIAN_POINT ( 'NONE',  ( -4.999999999999998224, -44.99999999999997158, -96.49999999781503845 ) ) ;
#3268=CARTESIAN_POINT ( 'NONE',  ( -4.566987299999998307, -43.10829192115428299, -99.29999999890752349 ) ) ;
#3269=CARTESIAN_POINT ( 'NONE',  ( -4.864554114591847167, -46.28939218662745247, -100.0008501927092226 ) ) ;
#3272=EDGE_CURVE ( 'NONE', #2422, #5583, #3112, .T. ) ;
#3273=VECTOR ( 'NONE', #7798, 1000.000000000000000 ) ;
#3274=CARTESIAN_POINT ( 'NONE',  ( -4.999999999999997335, -47.07106781186546129, -97.34300000002184561 ) ) ;
#3287=CARTESIAN_POINT ( 'NONE',  ( -4.566987299999998307, -44.99999999999997158, -95.34999999890753486 ) ) ;
#3293=CARTESIAN_POINT ( 'NONE',  ( -3.061616997868382155E-16, -39.99999999999997158, -100.6999999978150555 ) ) ;
#3294=CARTESIAN_POINT ( 'NONE',  ( -1.891708078845683039, -40.43301269999998482, -100.3999999989075178 ) ) ;
#3304=CARTESIAN_POINT ( 'NONE',  ( 4.999999999999998224, -42.92893218813449607, -99.35000000000000853 ) ) ;
#3305=CARTESIAN_POINT ( 'NONE',  ( -4.999999999999998224, -44.99999999999997158, -98.89999999781504414 ) ) ;
#3307=CARTESIAN_POINT ( 'NONE',  ( -3.535533905932735532, -48.53553390593270933, -99.70000000000000284 ) ) ;
#3313=CARTESIAN_POINT ( 'NONE',  ( -2.796473189345805913E-16, -40.43301269999997061, -98.84999999890752065 ) ) ;
#3314=CARTESIAN_POINT ( 'NONE',  ( 2.071067811865474173, -39.99999999999997158, -96.74999999781503845 ) ) ;
#3316=CARTESIAN_POINT ( 'NONE',  ( 8.389419568037416259E-16, -49.56698729999997255, -97.44999999890751496 ) ) ;
#3317=CARTESIAN_POINT ( 'NONE',  ( 5.007363570061430735, -45.07891398322220056, -99.99974818118526798 ) ) ;
#3319=CARTESIAN_POINT ( 'NONE',  ( -4.999999999999998224, -45.95670858091268940, -94.96990301170907856 ) ) ;
#3329=CARTESIAN_POINT ( 'NONE',  ( -4.999999999999998224, -44.99999999999997158, -99.00000000000000000 ) ) ;
#3333=CARTESIAN_POINT ( 'NONE',  ( 1.891708078845682595, -40.43301269999998482, -95.49999999890754054 ) ) ;
#3335=ORIENTED_EDGE ( 'NONE', *, *, #2748, .F. ) ;
#3345=CARTESIAN_POINT ( 'NONE',  ( -3.061616997868382155E-16, -39.99999999999997158, -99.20000000000000284 ) ) ;
#3346=CARTESIAN_POINT ( 'NONE',  ( 4.999999999999998224, -42.92893218813448897, -100.0499999978150356 ) ) ;
#3348=CARTESIAN_POINT ( 'NONE',  ( 4.999999999999998224, -44.99999999999997158, -98.60000000000000853 ) ) ;
#3356=CARTESIAN_POINT ( 'NONE',  ( -4.566987299999998307, -44.99999999999997158, -98.64999999890751781 ) ) ;
#3357=CARTESIAN_POINT ( 'NONE',  ( -3.535533905932735532, -48.53553390593270933, -99.70000000000000284 ) ) ;
#3359=CARTESIAN_POINT ( 'NONE',  ( 4.566987300000000083, -46.89170807884565306, -98.89999999890753202 ) ) ;
#3363=CARTESIAN_POINT ( 'NONE',  ( 2.071067811865474173, -39.99999999999997158, -96.84300000002187403 ) ) ;
#3365=CARTESIAN_POINT ( 'NONE',  ( 2.071067811865474173, -39.99999999999997158, -97.65000000000000568 ) ) ;
#3369=CARTESIAN_POINT ( 'NONE',  ( -5.000000000000007105, -47.07106781186543998, -99.74999999999998579 ) ) ;
#3372=CARTESIAN_POINT ( 'NONE',  ( -4.999999999999998224, -44.99999999999997158, -96.60000000000000853 ) ) ;
#3378=CARTESIAN_POINT ( 'NONE',  ( -2.796473189345805913E-16, -40.43301269999997061, -96.24999999890752633 ) ) ;
#3388=CARTESIAN_POINT ( 'NONE',  ( -2.796473189345805913E-16, -40.43301269999997061, -100.2499999989075263 ) ) ;
#3389=CARTESIAN_POINT ( 'NONE',  ( 4.999999999999998224, -44.99999999999997158, -99.40000000000000568 ) ) ;
#3391=CARTESIAN_POINT ( 'NONE',  ( 2.071067811865474173, -39.99999999999997158, -98.34999999781506119 ) ) ;
#3393=CARTESIAN_POINT ( 'NONE',  ( 9.184850993605145972E-16, -49.99999999999997158, -99.59999999999999432 ) ) ;
#3399=CARTESIAN_POINT ( 'NONE',  ( 1.891708078845685481, -49.56698729999997255, -97.59999999890753486 ) ) ;
#3400=CARTESIAN_POINT ( 'NONE',  ( -4.999999999999998224, -42.92893218813448897, -96.54999999781504982 ) ) ;
#3402=CARTESIAN_POINT ( 'NONE',  ( 1.891708078845682595, -40.43301269999998482, -97.89999999890753202 ) ) ;
#3406=CARTESIAN_POINT ( 'NONE',  ( 4.999999999999998224, -44.99999999999997158, -96.99300000002185129 ) ) ;
#3410=CARTESIAN_POINT ( 'NONE',  ( 2.071067811865474173, -39.99999999999997158, -95.94999999781504130 ) ) ;
#3436=CARTESIAN_POINT ( 'NONE',  ( 4.566987299999998307, -43.10829192115428299, -95.79999999890752349 ) ) ;
#3442=ORIENTED_EDGE ( 'NONE', *, *, #6773, .T. ) ;
#3444=CARTESIAN_POINT ( 'NONE',  ( -2.796473189345805913E-16, -40.43301269999997061, -96.44999999890751496 ) ) ;
#3446=CARTESIAN_POINT ( 'NONE',  ( -3.061616997868382155E-16, -39.99999999999997158, -96.69999999781504130 ) ) ;
#3448=CARTESIAN_POINT ( 'NONE',  ( 4.566987299999998307, -44.99999999999997158, -98.04999999890752349 ) ) ;
#3452=CARTESIAN_POINT ( 'NONE',  ( -3.535533905932735532, -48.53553390593270933, -96.49300000002185129 ) ) ;
#3469=CIRCLE ( 'NONE', #5012, 4.999999999999998224 ) ;
#3476=CARTESIAN_POINT ( 'NONE',  ( -4.566987299999998307, -43.10829192115428299, -95.29999999890752349 ) ) ;
#3478=CARTESIAN_POINT ( 'NONE',  ( -3.229347689422839451, -48.22934768942280925, -98.54999999890752349 ) ) ;
#3479=CARTESIAN_POINT ( 'NONE',  ( 0.000000000000000000, -44.99999999999997158, -105.0000000000000142 ) ) ;
#3480=CARTESIAN_POINT ( 'NONE',  ( -4.999999999999998224, -44.99999999999997158, -96.49999999781503845 ) ) ;
#3488=CARTESIAN_POINT ( 'NONE',  ( -1.891708078845683705, -49.56698729999997255, -96.89999999890753202 ) ) ;
#3489=CARTESIAN_POINT ( 'NONE',  ( -4.999999999999998224, -42.92893218813448897, -100.5499999978150498 ) ) ;
#3491=CARTESIAN_POINT ( 'NONE',  ( 3.229347689422841228, -48.22934768942280925, -97.34999999890753486 ) ) ;
#3496=CARTESIAN_POINT ( 'NONE',  ( -3.535533905932736864, -41.46446609406723383, -95.10000000000000853 ) ) ;
#3499=( BOUNDED_SURFACE ( )  B_SPLINE_SURFACE ( 1, 2, ( 
 ( #5071, #7055, #2310, #8390, #5776, #7671, #547, #3256, #4944, #6306, #5031, #8343, #5643, #2262, #1774, #2351, #2968, #7624, #8472, #311, #6347, #1589, #3013, #348, #7762, #930, #7809, #3056, #1634, #8301, #7721, #5688, #389, #5733, #1729, #4328, #3623, #4370, #1015, #7009, #972, #4455, #6391, #3667, #4415, #7101, #1058, #3751, #6436, #2435, #4708, #8013, #5267, #3391, #2685, #1258, #5979, #26, #592, #5352, #4749, #775, #2064, #5397, #3305, #6814, #6067, #2727, #1346, #7477, #2641, #1440, #6633, #1931, #8672, #5312, #5937, #4133, #8106, #1970, #5440, #8055, #7968, #4045, #6765, #2112, #4658, #3346, #2598, #6023, #4617, #8712, #7346, #3956, #8631, #2019, #729, #6726, #7392, #7301, #1302 ),
 ( #685, #4001, #6681, #7436, #1393, #639, #4089, #3436, #6111, #68, #2775, #8153, #4794, #8196, #5575, #5010, #2816, #2156, #245, #4841, #6160, #7699, #289, #4967, #4262, #4174, #117, #4883, #2244, #7604, #6900, #6856, #7520, #1659, #908, #1613, #2860, #1523, #821, #5488, #1480, #8369, #6987, #2331, #1566, #4923, #951, #4350, #3603, #5535, #6324, #3521, #861, #6944, #6284, #6247, #6199, #3646, #2990, #2946, #7030, #5666, #3478, #163, #8240, #2198, #5621, #7561, #4217, #8323, #3563, #2285, #204, #2906, #8283, #7650, #4302, #8529, #8489, #6369, #4435, #5093, #3814, #1833, #4515, #7827, #2415, #5710, #3118, #2536, #330, #8412, #6495, #2376, #3689, #5215, #6537, #2495, #1792, #1704, #3036 ) ),
 .UNSPECIFIED., .F., .F., .T. ) 
 B_SPLINE_SURFACE_WITH_KNOTS ( ( 2, 2 ),
 ( 3, 2, 2, 2, 2, 2, 2, 2, 2, 2, 2, 2, 2, 2, 2, 2, 2, 2, 2, 2, 2, 2, 2, 2, 2, 2, 2, 2, 2, 2, 2, 2, 2, 2, 2, 2, 2, 2, 2, 2, 2, 2, 2, 2, 2, 2, 2, 2, 2, 2, 3 ),
 ( 0.000000000000000000, 1.000000000000000000 ),
 ( 0.000000000000000000, 0.01785714285714285615, 0.03571428571428571230, 0.05357142857142856845, 0.07142857142857142461, 0.08928571428571428770, 0.1071428571428571369, 0.1250000000000000000, 0.1428571428571428492, 0.1607142857142857262, 0.1785714285714285754, 0.1964285714285714246, 0.2142857142857142738, 0.2321428571428571508, 0.2500000000000000000, 0.2678571428571428492, 0.2857142857142856984, 0.3035714285714285476, 0.3214285714285714524, 0.3392857142857143016, 0.3571428571428571508, 0.3750000000000000000, 0.3928571428571428492, 0.4107142857142856984, 0.4285714285714285476, 0.4464285714285714524, 0.4642857142857143016, 0.4821428571428571508, 0.5000000000000000000, 0.5178571428571429047, 0.5357142857142856984, 0.5535714285714286031, 0.5714285714285713969, 0.5892857142857143016, 0.6071428571428570953, 0.6250000000000000000, 0.6428571428571429047, 0.6607142857142856984, 0.6785714285714286031, 0.6964285714285713969, 0.7142857142857143016, 0.7321428571428570953, 0.7500000000000000000, 0.7678571428571429047, 0.7857142857142856984, 0.8035714285714286031, 0.8214285714285713969, 0.8392857142857143016, 0.8571428571428570953, 0.8750000000000000000, 0.8928571428571429047 ),
 .UNSPECIFIED. ) 
 GEOMETRIC_REPRESENTATION_ITEM ( )  RATIONAL_B_SPLINE_SURFACE ( (
 ( 1.000000000000000000, 0.9238795325112867385, 1.000000000000000000, 0.9238795325112867385, 1.000000000000000000, 0.9238795325112867385, 1.000000000000000000, 0.9238795325112867385, 1.000000000000000000, 0.9238795325112867385, 1.000000000000000000, 0.9238795325112867385, 1.000000000000000000, 0.9238795325112867385, 1.000000000000000000, 0.9238795325112867385, 1.000000000000000000, 0.9238795325112867385, 1.000000000000000000, 0.9238795325112867385, 1.000000000000000000, 0.9238795325112867385, 1.000000000000000000, 0.9238795325112867385, 1.000000000000000000, 0.9238795325112867385, 1.000000000000000000, 0.9238795325112867385, 1.000000000000000000, 0.9238795325112867385, 1.000000000000000000, 0.9238795325112867385, 1.000000000000000000, 0.9238795325112867385, 1.000000000000000000, 0.9238795325112867385, 1.000000000000000000, 0.9238795325112867385, 1.000000000000000000, 0.9238795325112867385, 1.000000000000000000, 0.9238795325112867385, 1.000000000000000000, 0.9238795325112867385, 1.000000000000000000, 0.9238795325112867385, 1.000000000000000000, 0.9238795325112867385, 1.000000000000000000, 0.9238795325112867385, 1.000000000000000000, 0.9238795325112867385, 1.000000000000000000, 0.9238795325112867385, 1.000000000000000000, 0.9238795325112867385, 1.000000000000000000, 0.9238795325112867385, 1.000000000000000000, 0.9238795325112867385, 1.000000000000000000, 0.9238795325112867385, 1.000000000000000000, 0.9238795325112867385, 1.000000000000000000, 0.9238795325112867385, 1.000000000000000000, 0.9238795325112867385, 1.000000000000000000, 0.9238795325112867385, 1.000000000000000000, 0.9238795325112867385, 1.000000000000000000, 0.9238795325112867385, 1.000000000000000000, 0.9238795325112867385, 1.000000000000000000, 0.9238795325112867385, 1.000000000000000000, 0.9238795325112867385, 1.000000000000000000, 0.9238795325112867385, 1.000000000000000000, 0.9238795325112867385, 1.000000000000000000, 0.9238795325112867385, 1.000000000000000000, 0.9238795325112867385, 1.000000000000000000, 0.9238795325112867385, 1.000000000000000000, 0.9238795325112867385, 1.000000000000000000, 0.9238795325112867385, 1.000000000000000000, 0.9238795325112867385, 1.000000000000000000, 0.9238795325112867385, 1.000000000000000000, 0.9238795325112867385, 1.000000000000000000),
 ( 1.000000000000000000, 0.9238795325112867385, 1.000000000000000000, 0.9238795325112867385, 1.000000000000000000, 0.9238795325112867385, 1.000000000000000000, 0.9238795325112867385, 1.000000000000000000, 0.9238795325112867385, 1.000000000000000000, 0.9238795325112867385, 1.000000000000000000, 0.9238795325112867385, 1.000000000000000000, 0.9238795325112867385, 1.000000000000000000, 0.9238795325112867385, 1.000000000000000000, 0.9238795325112867385, 1.000000000000000000, 0.9238795325112867385, 1.000000000000000000, 0.9238795325112867385, 1.000000000000000000, 0.9238795325112867385, 1.000000000000000000, 0.9238795325112867385, 1.000000000000000000, 0.9238795325112867385, 1.000000000000000000, 0.9238795325112867385, 1.000000000000000000, 0.9238795325112867385, 1.000000000000000000, 0.9238795325112867385, 1.000000000000000000, 0.9238795325112867385, 1.000000000000000000, 0.9238795325112867385, 1.000000000000000000, 0.9238795325112867385, 1.000000000000000000, 0.9238795325112867385, 1.000000000000000000, 0.9238795325112867385, 1.000000000000000000, 0.9238795325112867385, 1.000000000000000000, 0.9238795325112867385, 1.000000000000000000, 0.9238795325112867385, 1.000000000000000000, 0.9238795325112867385, 1.000000000000000000, 0.9238795325112867385, 1.000000000000000000, 0.9238795325112867385, 1.000000000000000000, 0.9238795325112867385, 1.000000000000000000, 0.9238795325112867385, 1.000000000000000000, 0.9238795325112867385, 1.000000000000000000, 0.9238795325112867385, 1.000000000000000000, 0.9238795325112867385, 1.000000000000000000, 0.9238795325112867385, 1.000000000000000000, 0.9238795325112867385, 1.000000000000000000, 0.9238795325112867385, 1.000000000000000000, 0.9238795325112867385, 1.000000000000000000, 0.9238795325112867385, 1.000000000000000000, 0.9238795325112867385, 1.000000000000000000, 0.9238795325112867385, 1.000000000000000000, 0.9238795325112867385, 1.000000000000000000, 0.9238795325112867385, 1.000000000000000000, 0.9238795325112867385, 1.000000000000000000, 0.9238795325112867385, 1.000000000000000000, 0.9238795325112867385, 1.000000000000000000, 0.9238795325112867385, 1.000000000000000000, 0.9238795325112867385, 1.000000000000000000, 0.9238795325112867385, 1.000000000000000000, 0.9238795325112867385, 1.000000000000000000) ) ) 
 REPRESENTATION_ITEM ( '' )  SURFACE ( )  );
#3510=CARTESIAN_POINT ( 'NONE',  ( -4.999999999999997335, -47.07106781186546129, -99.64999999781505835 ) ) ;
#3518=CARTESIAN_POINT ( 'NONE',  ( 4.566987299999998307, -44.99999999999997158, -97.24999999890752633 ) ) ;
#3521=CARTESIAN_POINT ( 'NONE',  ( -1.891708078845683039, -40.43301269999998482, -97.99999999890752633 ) ) ;
#3530=CARTESIAN_POINT ( 'NONE',  ( 4.999999999999998224, -44.99999999999997158, -98.49999999781503845 ) ) ;
#3531=CARTESIAN_POINT ( 'NONE',  ( -2.071067811865475061, -39.99999999999997158, -98.24999999781505267 ) ) ;
#3532=CARTESIAN_POINT ( 'NONE',  ( 3.535533905932737309, -48.53553390593270933, -98.59999999781504698 ) ) ;
#3533=CARTESIAN_POINT ( 'NONE',  ( 4.999999999999998224, -44.99999999999997158, -97.69999999781505551 ) ) ;
#3534=CARTESIAN_POINT ( 'NONE',  ( -4.566987299999998307, -43.10829192115428299, -97.69999999890751496 ) ) ;
#3537=CARTESIAN_POINT ( 'NONE',  ( -4.999999999999998224, -44.99999999999997158, -95.00000000000000000 ) ) ;
#3539=CARTESIAN_POINT ( 'NONE',  ( 4.566987300000000083, -46.89170807884565306, -96.49999999890752633 ) ) ;
#3558=ORIENTED_EDGE ( 'NONE', *, *, #2044, .T. ) ;
#3559=CARTESIAN_POINT ( 'NONE',  ( -1.891708078845683039, -40.43301269999998482, -95.39999999890753202 ) ) ;
#3563=CARTESIAN_POINT ( 'NONE',  ( 3.229347689422839895, -41.77065231057713390, -98.94999999890752918 ) ) ;
#3575=CARTESIAN_POINT ( 'NONE',  ( 2.071067811865477282, -49.99999999999996447, -100.2499999978150669 ) ) ;
#3577=CARTESIAN_POINT ( 'NONE',  ( -4.566987299999998307, -43.10829192115428299, -98.49999999890752633 ) ) ;
#3581=CARTESIAN_POINT ( 'NONE',  ( -2.071067811865475505, -49.99999999999996447, -98.84300000002188824 ) ) ;
#3582=FACE_OUTER_BOUND ( 'NONE', #5975, .T. ) ;
#3593=CARTESIAN_POINT ( 'NONE',  ( 4.999999999999998224, -44.99999999999997158, -97.79999999999999716 ) ) ;
#3601=CARTESIAN_POINT ( 'NONE',  ( 1.891708078845682595, -40.43301269999998482, -97.09999999890753486 ) ) ;
#3603=CARTESIAN_POINT ( 'NONE',  ( -4.566987299999998307, -44.99999999999997158, -97.84999999890752065 ) ) ;
#3606=CARTESIAN_POINT ( 'NONE',  ( 2.071067811865477282, -49.99999999999997158, -96.24999999781505267 ) ) ;
#3613=CARTESIAN_POINT ( 'NONE',  ( -4.999999999999997335, -47.07106781186546129, -98.84999999781503277 ) ) ;
#3616=CARTESIAN_POINT ( 'NONE',  ( -3.061616997868382155E-16, -39.99999999999997158, -98.29999999781504982 ) ) ;
#3618=CARTESIAN_POINT ( 'NONE',  ( -4.566987299999998307, -44.99999999999997158, -100.0499999989075235 ) ) ;
#3621=CARTESIAN_POINT ( 'NONE',  ( 1.932551333443697450, -39.99999999999997158, -100.0396559164136931 ) ) ;
#3622=CARTESIAN_POINT ( 'NONE',  ( 3.229347689422841228, -48.22934768942280925, -95.74999999890752633 ) ) ;
#3623=CARTESIAN_POINT ( 'NONE',  ( -3.061616997868382155E-16, -39.99999999999997158, -97.49999999781503845 ) ) ;
#3629=LINE ( 'NONE', #3222, #8256 ) ;
#3632=CARTESIAN_POINT ( 'NONE',  ( 0.6544984694978718265, -39.99999999999997868, -100.0000000000000142 ) ) ;
#3643=CARTESIAN_POINT ( 'NONE',  ( 4.566987299999998307, -44.99999999999997158, -96.44999999890752918 ) ) ;
#3646=CARTESIAN_POINT ( 'NONE',  ( 4.566987300000000083, -46.89170807884565306, -98.29999999890752349 ) ) ;
#3648=CARTESIAN_POINT ( 'NONE',  ( 3.229347689422839895, -41.77065231057713390, -95.74999999890751212 ) ) ;
#3658=CARTESIAN_POINT ( 'NONE',  ( -4.999999999999998224, -42.92893218813448897, -98.14999999781504414 ) ) ;
#3661=CARTESIAN_POINT ( 'NONE',  ( -3.535533905932735532, -48.53553390593270933, -95.70000000000000284 ) ) ;
#3665=CARTESIAN_POINT ( 'NONE',  ( -2.071067811865475505, -49.99999999999996447, -99.64300000002187119 ) ) ;
#3666=CARTESIAN_POINT ( 'NONE',  ( -4.566987299999998307, -43.10829192115428299, -95.29999999890750928 ) ) ;
#3667=CARTESIAN_POINT ( 'NONE',  ( 2.071067811865477282, -49.99999999999996447, -97.84999999781504698 ) ) ;
#3671=PRODUCT ( 'position indicator', 'position indicator', '', ( #5510 ) ) ;
#3686=CARTESIAN_POINT ( 'NONE',  ( -2.796473189345805913E-16, -40.43301269999997061, -100.2499999989075263 ) ) ;
#3689=CARTESIAN_POINT ( 'NONE',  ( -3.229347689422839451, -48.22934768942280925, -100.1499999989075178 ) ) ;
#3691=CARTESIAN_POINT ( 'NONE',  ( 4.566987299999998307, -43.10829192115428299, -98.19999999890751496 ) ) ;
#3692=DIRECTION ( 'NONE',  ( 1.000000000000000000, 0.000000000000000000, 0.000000000000000000 ) ) ;
#3703=CARTESIAN_POINT ( 'NONE',  ( 2.071067811865474173, -39.99999999999997158, -95.25000000000000000 ) ) ;
#3705=ADVANCED_BREP_SHAPE_REPRESENTATION ( '', ( #8634, #2554 ), #564 ) ;
#3709=CARTESIAN_POINT ( 'NONE',  ( -4.566987299999998307, -43.10829192115428299, -96.09999999890752065 ) ) ;
#3715=CARTESIAN_POINT ( 'NONE',  ( 8.389419568037416259E-16, -49.56698729999997255, -96.04999999890752349 ) ) ;
#3720=FACE_OUTER_BOUND ( 'NONE', #200, .T. ) ;
#3722=EDGE_LOOP ( 'NONE', ( #3335, #1556, #6761, #7430 ) ) ;
#3727=( BOUNDED_CURVE ( )  B_SPLINE_CURVE ( 2, ( #472, #4544, #7938, #4376, #4499, #5198, #5121, #354, #7230 ),
 .UNSPECIFIED., .F., .T. ) 
 B_SPLINE_CURVE_WITH_KNOTS ( ( 3, 2, 2, 2, 3 ),
 ( 0.2142857142857142738, 0.2321428571428571508, 0.2500000000000000000, 0.2678571428571428492, 0.2857142857142856984 ),
 .UNSPECIFIED. ) 
 CURVE ( )  GEOMETRIC_REPRESENTATION_ITEM ( )  RATIONAL_B_SPLINE_CURVE ( ( 1.000000000000000000, 0.9238795325112867385, 1.000000000000000000, 0.9238795325112867385, 1.000000000000000000, 0.9238795325112867385, 1.000000000000000000, 0.9238795325112867385, 1.000000000000000000 ) ) 
 REPRESENTATION_ITEM ( '' )  );
#3728=CARTESIAN_POINT ( 'NONE',  ( -3.229347689422840784, -41.77065231057713390, -98.54999999890752349 ) ) ;
#3733=CARTESIAN_POINT ( 'NONE',  ( -3.229347689422840784, -41.77065231057713390, -97.94999999890751496 ) ) ;
#3742=CARTESIAN_POINT ( 'NONE',  ( 4.999999999999998224, -44.99999999999997158, -97.69999999781505551 ) ) ;
#3744=CARTESIAN_POINT ( 'NONE',  ( -4.999999999999997335, -47.07106781186546129, -96.54999999999999716 ) ) ;
#3750=CARTESIAN_POINT ( 'NONE',  ( -4.999999999999998224, -42.92893218813448897, -96.64999999999999147 ) ) ;
#3751=CARTESIAN_POINT ( 'NONE',  ( -4.999999999999997335, -47.07106781186546129, -98.04999999781504982 ) ) ;
#3757=CARTESIAN_POINT ( 'NONE',  ( 3.535533905932736420, -41.46446609406723383, -98.50000000000000000 ) ) ;
#3771=CARTESIAN_POINT ( 'NONE',  ( 1.891708078845685481, -49.56698729999997255, -99.79999999890752349 ) ) ;
#3776=CARTESIAN_POINT ( 'NONE',  ( -3.229347689422839451, -48.22934768942280925, -97.74999999890751212 ) ) ;
#3781=( BOUNDED_CURVE ( )  B_SPLINE_CURVE ( 2, ( #502, #3132, #2511, #3214, #5811, #2466, #5898, #5148, #1133 ),
 .UNSPECIFIED., .F., .T. ) 
 B_SPLINE_CURVE_WITH_KNOTS ( ( 3, 2, 2, 2, 3 ),
 ( 0.3571428571428570953, 0.3750000000000000000, 0.3928571428571428492, 0.4107142857142856984, 0.4285714285714286031 ),
 .UNSPECIFIED. ) 
 CURVE ( )  GEOMETRIC_REPRESENTATION_ITEM ( )  RATIONAL_B_SPLINE_CURVE ( ( 1.000000000000000222, 0.9238795325112865164, 1.000000000000000000, 0.9238795325112867385, 1.000000000000000000, 0.9238795325112867385, 1.000000000000000000, 0.9238795325112865164, 1.000000000000000222 ) ) 
 REPRESENTATION_ITEM ( '' )  );
#3784=ORIENTED_EDGE ( 'NONE', *, *, #2203, .T. ) ;
#3786=FACE_OUTER_BOUND ( 'NONE', #1031, .T. ) ;
#3788=CARTESIAN_POINT ( 'NONE',  ( 9.184850993605145972E-16, -49.99999999999997158, -95.60000000000000853 ) ) ;
#3790=CARTESIAN_POINT ( 'NONE',  ( -2.071067811865475061, -39.99999999999997158, -96.75000000000001421 ) ) ;
#3794=CARTESIAN_POINT ( 'NONE',  ( -2.071067811865475505, -49.99999999999996447, -97.25000000000000000 ) ) ;
#3795=CARTESIAN_POINT ( 'NONE',  ( -2.740268896160362289, -40.77945301579084969, -99.99896619294457878 ) ) ;
#3801=CYLINDRICAL_SURFACE ( 'NONE', #7714, 4.999999999999998224 ) ;
#3803=B_SPLINE_CURVE_WITH_KNOTS ( 'NONE', 3,
 ( #3226, #3969, #5863, #558, #3795, #6562, #1858, #8682, #4456, #3183, #3927, #514, #6647, #6602, #8597, #3269, #1814, #5118, #603, #5950, #7810, #5908, #6475, #8643, #2609, #5157, #6517, #7142, #5277, #7225, #427, #8555, #2562, #2519, #3143, #5240, #7183, #2475, #7934, #3317, #7982, #1943, #1269, #1103, #5195, #5823 ),
 .UNSPECIFIED., .F., .F.,
 ( 4, 2, 2, 2, 2, 2, 2, 2, 2, 2, 2, 2, 2, 2, 2, 2, 2, 2, 2, 2, 2, 2, 4 ),
 ( 0.000000000000000000, 0.06249999999999973632, 0.1249999999999994726, 0.1562499999999996114, 0.1874999999999997780, 0.2500000000000000555, 0.2812499999999998335, 0.3124999999999995559, 0.3749999999999990563, 0.4062499999999988343, 0.4374999999999986122, 0.4999999999999986677, 0.5624999999999987788, 0.5937499999999987788, 0.6249999999999988898, 0.6874999999999992228, 0.7187499999999993339, 0.7499999999999993339, 0.8124999999999995559, 0.8437499999999996669, 0.8749999999999997780, 0.9374999999999998890, 1.000000000000000000 ),
 .UNSPECIFIED. ) ;
#3814=CARTESIAN_POINT ( 'NONE',  ( -3.229347689422840784, -41.77065231057713390, -99.54999999890752349 ) ) ;
#3816=CARTESIAN_POINT ( 'NONE',  ( 4.566987299999998307, -44.99999999999997158, -95.84999999890752065 ) ) ;
#3830=CARTESIAN_POINT ( 'NONE',  ( -3.061616997868382155E-16, -39.99999999999997158, -95.20000000000000284 ) ) ;
#3833=ORIENTED_EDGE ( 'NONE', *, *, #701, .T. ) ;
#3834=CARTESIAN_POINT ( 'NONE',  ( 3.535533905932737309, -48.53553390593270933, -96.29999999999999716 ) ) ;
#3851=ADVANCED_FACE ( 'NONE', ( #102 ), #189, .T. ) ;
#3853=CARTESIAN_POINT ( 'NONE',  ( 4.566987300000000083, -46.89170807884564596, -98.09999999890753486 ) ) ;
#3860=CARTESIAN_POINT ( 'NONE',  ( 4.566987300000000083, -46.89170807884565306, -95.69999999890755760 ) ) ;
#3862=EDGE_LOOP ( 'NONE', ( #5494, #7552, #4570, #75 ) ) ;
#3880=CARTESIAN_POINT ( 'NONE',  ( -4.999999999999997335, -47.07106781186546129, -96.54999999999999716 ) ) ;
#3884=CARTESIAN_POINT ( 'NONE',  ( -3.061616997868382155E-16, -39.99999999999997158, -99.89999999781504414 ) ) ;
#3903=CARTESIAN_POINT ( 'NONE',  ( 4.566987299999998307, -43.10829192115428299, -99.79999999890752349 ) ) ;
#3924=CARTESIAN_POINT ( 'NONE',  ( 5.000000000000000000, -47.07106781186545419, -99.45000000000000284 ) ) ;
#3926=CARTESIAN_POINT ( 'NONE',  ( 4.566987300000000083, -46.89170807884565306, -99.69999999890752918 ) ) ;
#3927=CARTESIAN_POINT ( 'NONE',  ( -4.794783009932419127, -43.47026749230783338, -99.99939984573538254 ) ) ;
#3930=CARTESIAN_POINT ( 'NONE',  ( 3.535533905932737309, -48.53553390593270933, -96.29300000002184845 ) ) ;
#3942=DIRECTION ( 'NONE',  ( 0.000000000000000000, 0.000000000000000000, 1.000000000000000000 ) ) ;
#3945=CARTESIAN_POINT ( 'NONE',  ( -4.566987299999998307, -43.10829192115428299, -99.49999999890754054 ) ) ;
#3947=ORIENTED_EDGE ( 'NONE', *, *, #793, .T. ) ;
#3948=CARTESIAN_POINT ( 'NONE',  ( -7.499999999999999112, -44.99999999999997158, -105.0000000000000142 ) ) ;
#3956=CARTESIAN_POINT ( 'NONE',  ( -2.071067811865475505, -49.99999999999996447, -100.3499999978150754 ) ) ;
#3957=CARTESIAN_POINT ( 'NONE',  ( -4.999999999999998224, -44.99999999999997158, -95.00000000000000000 ) ) ;
#3958=CARTESIAN_POINT ( 'NONE',  ( -4.999999999999997335, -47.07106781186546129, -99.75000000000001421 ) ) ;
#3962=( GEOMETRIC_REPRESENTATION_CONTEXT ( 3 ) GLOBAL_UNCERTAINTY_ASSIGNED_CONTEXT ( ( #8388 ) ) GLOBAL_UNIT_ASSIGNED_CONTEXT ( ( #4077, #149, #2186 ) ) REPRESENTATION_CONTEXT ( 'NONE', 'WORKASPACE' ) );
#3963=EDGE_CURVE ( 'NONE', #5746, #1056, #3238, .T. ) ;
#3965=CARTESIAN_POINT ( 'NONE',  ( -3.229347689422839451, -48.22934768942280925, -98.54999999890752349 ) ) ;
#3966=CARTESIAN_POINT ( 'NONE',  ( 3.535533905932737309, -48.53553390593270933, -96.19999999781504130 ) ) ;
#3968=CARTESIAN_POINT ( 'NONE',  ( 8.389419568037416259E-16, -49.56698729999997255, -99.84999999890753486 ) ) ;
#3969=CARTESIAN_POINT ( 'NONE',  ( -0.5580800036469334424, -39.99999999999998579, -100.0011100901508883 ) ) ;
#3972=CARTESIAN_POINT ( 'NONE',  ( -3.535533905932736864, -41.46446609406723383, -96.69300000002185413 ) ) ;
#3978=ORIENTED_EDGE ( 'NONE', *, *, #486, .F. ) ;
#3983=CARTESIAN_POINT ( 'NONE',  ( -3.061616997868382155E-16, -39.99999999999997158, -96.79999999999999716 ) ) ;
#3989=CARTESIAN_POINT ( 'NONE',  ( -1.891708078845683039, -40.43301269999998482, -95.39999999890751781 ) ) ;
#3991=ORIENTED_EDGE ( 'NONE', *, *, #3113, .F. ) ;
#3997=EDGE_LOOP ( 'NONE', ( #4220, #6405, #2644, #1979 ) ) ;
#4001=CARTESIAN_POINT ( 'NONE',  ( -4.566987299999998307, -43.10829192115428299, -95.49999999890754054 ) ) ;
#4003=CARTESIAN_POINT ( 'NONE',  ( -3.061616997868382155E-16, -39.99999999999997158, -99.20000000000000284 ) ) ;
#4004=CIRCLE ( 'NONE', #6104, 7.499999999999999112 ) ;
#4008=( BOUNDED_CURVE ( )  B_SPLINE_CURVE ( 2, ( #4684, #7370, #4025, #1908, #6702, #4773, #2706, #3369, #4595 ),
 .UNSPECIFIED., .F., .T. ) 
 B_SPLINE_CURVE_WITH_KNOTS ( ( 3, 2, 2, 2, 3 ),
 ( 0.7857142857142856984, 0.8035714285714286031, 0.8214285714285713969, 0.8392857142857144126, 0.8571428571428572063 ),
 .UNSPECIFIED. ) 
 CURVE ( )  GEOMETRIC_REPRESENTATION_ITEM ( )  RATIONAL_B_SPLINE_CURVE ( ( 1.000000000000000000, 0.9238795325112867385, 1.000000000000000000, 0.9238795325112867385, 1.000000000000000000, 0.9238795325112867385, 1.000000000000000000, 0.9238795325112862944, 1.000000000000000444 ) ) 
 REPRESENTATION_ITEM ( '' )  );
#4010=CARTESIAN_POINT ( 'NONE',  ( 8.389419568037416259E-16, -49.56698729999997255, -99.24999999890751212 ) ) ;
#4011=CARTESIAN_POINT ( 'NONE',  ( -4.999999999999998224, -42.92893218813448897, -97.34999999781506119 ) ) ;
#4013=CARTESIAN_POINT ( 'NONE',  ( -1.891708078845683039, -40.43301269999998482, -97.79999999890752349 ) ) ;
#4017=CARTESIAN_POINT ( 'NONE',  ( 2.071067811865474173, -39.99999999999997158, -97.64300000002185698 ) ) ;
#4024=ORIENTED_EDGE ( 'NONE', *, *, #6419, .F. ) ;
#4025=CARTESIAN_POINT ( 'NONE',  ( 3.535533905932737309, -48.53553390593270933, -99.50000000000000000 ) ) ;
#4034=CARTESIAN_POINT ( 'NONE',  ( -1.891708078845683483, -49.56698729999997255, -99.29999999890752349 ) ) ;
#4037=EDGE_CURVE ( 'NONE', #799, #2422, #2883, .T. ) ;
#4045=CARTESIAN_POINT ( 'NONE',  ( -2.071067811865475061, -39.99999999999997158, -99.84999999781504698 ) ) ;
#4046=CARTESIAN_POINT ( 'NONE',  ( 5.000000000000000000, -47.07106781186545419, -96.25000000000000000 ) ) ;
#4047=CARTESIAN_POINT ( 'NONE',  ( 5.000000000000000000, -47.07106781186545419, -98.65000000000000568 ) ) ;
#4054=CARTESIAN_POINT ( 'NONE',  ( 4.566987300000000083, -46.89170807884564596, -98.29999999890752349 ) ) ;
#4056=CARTESIAN_POINT ( 'NONE',  ( 3.535533905932736420, -41.46446609406723383, -99.29999999999999716 ) ) ;
#4059=CARTESIAN_POINT ( 'NONE',  ( 4.566987299999998307, -43.10829192115428299, -97.99999999890754054 ) ) ;
#4063=CARTESIAN_POINT ( 'NONE',  ( -2.071067811865475061, -39.99999999999997158, -95.94300000002186835 ) ) ;
#4072=CARTESIAN_POINT ( 'NONE',  ( 4.999999999999998224, -44.99999999999997158, -96.20000000000000284 ) ) ;
#4073=DIRECTION ( 'NONE',  ( 0.000000000000000000, 0.000000000000000000, -1.000000000000000000 ) ) ;
#4077=( LENGTH_UNIT ( ) NAMED_UNIT ( * ) SI_UNIT ( .MILLI., .METRE. ) );
#4083=VERTEX_POINT ( 'NONE', #5827 ) ;
#4087=CARTESIAN_POINT ( 'NONE',  ( -4.999999999999998224, -44.99999999999997158, -99.00000000000000000 ) ) ;
#4089=CARTESIAN_POINT ( 'NONE',  ( 3.229347689422839895, -41.77065231057713390, -95.74999999890751212 ) ) ;
#4098=CARTESIAN_POINT ( 'NONE',  ( 4.566987299999998307, -44.99999999999997158, -96.64999999890753202 ) ) ;
#4099=CARTESIAN_POINT ( 'NONE',  ( 0.9662756667218486140, -39.99999999999997158, -100.0233279581959209 ) ) ;
#4101=CARTESIAN_POINT ( 'NONE',  ( 3.229347689422839895, -41.77065231057713390, -99.54999999890752349 ) ) ;
#4105=CARTESIAN_POINT ( 'NONE',  ( -2.071067811865475061, -39.99999999999997158, -95.14300000002184277 ) ) ;
#4131=CARTESIAN_POINT ( 'NONE',  ( 8.389419568037416259E-16, -49.56698729999997255, -96.64999999890753202 ) ) ;
#4133=CARTESIAN_POINT ( 'NONE',  ( -2.071067811865475505, -49.99999999999996447, -99.54999999781506403 ) ) ;
#4136=ORIENTED_EDGE ( 'NONE', *, *, #1709, .F. ) ;
#4141=ORIENTED_EDGE ( 'NONE', *, *, #2211, .F. ) ;
#4142=CARTESIAN_POINT ( 'NONE',  ( 2.071067811865477282, -49.99999999999997158, -98.64999999781504414 ) ) ;
#4143=CARTESIAN_POINT ( 'NONE',  ( -3.229347689422840784, -41.77065231057713390, -97.14999999890753202 ) ) ;
#4145=CARTESIAN_POINT ( 'NONE',  ( 4.999999999999998224, -44.99999999999997158, -99.29999999781504982 ) ) ;
#4147=CARTESIAN_POINT ( 'NONE',  ( -2.796473189345805913E-16, -40.43301269999997061, -97.84999999890753486 ) ) ;
#4148=FILL_AREA_STYLE ('',( #5324 ) ) ;
#4151=CARTESIAN_POINT ( 'NONE',  ( 2.071067811865477282, -49.99999999999996447, -98.74300000002187971 ) ) ;
#4163=( NAMED_UNIT ( * ) PLANE_ANGLE_UNIT ( ) SI_UNIT ( $, .RADIAN. ) );
#4165=CARTESIAN_POINT ( 'NONE',  ( -3.535533905932735532, -48.53553390593270933, -98.90000000000000568 ) ) ;
#4170=ADVANCED_FACE ( 'NONE', ( #7141 ), #3499, .T. ) ;
#4172=CARTESIAN_POINT ( 'NONE',  ( 3.229347689422841228, -48.22934768942280925, -95.74999999890752633 ) ) ;
#4174=CARTESIAN_POINT ( 'NONE',  ( 4.566987300000000083, -46.89170807884565306, -96.69999999890752918 ) ) ;
#4184=CARTESIAN_POINT ( 'NONE',  ( -4.566987299999998307, -44.99999999999997158, -99.44999999890752918 ) ) ;
#4186=CARTESIAN_POINT ( 'NONE',  ( 4.999999999999998224, -44.99999999999997158, -98.49999999781503845 ) ) ;
#4189=CARTESIAN_POINT ( 'NONE',  ( 3.229347689422839895, -41.77065231057713390, -99.54999999890752349 ) ) ;
#4191=CARTESIAN_POINT ( 'NONE',  ( -3.061616997868382155E-16, -39.99999999999997158, -96.00000000000000000 ) ) ;
#4192=CARTESIAN_POINT ( 'NONE',  ( 1.891708078845682595, -40.43301269999998482, -96.29999999890752349 ) ) ;
#4196=ORIENTED_EDGE ( 'NONE', *, *, #4705, .T. ) ;
#4197=CARTESIAN_POINT ( 'NONE',  ( -3.535533905932735532, -48.53553390593270933, -100.3999999978150441 ) ) ;
#4204=DIRECTION ( 'NONE',  ( 0.000000000000000000, 0.000000000000000000, -1.000000000000000000 ) ) ;
#4213=CARTESIAN_POINT ( 'NONE',  ( -4.566987299999998307, -44.99999999999997158, -96.84999999890753486 ) ) ;
#4217=CARTESIAN_POINT ( 'NONE',  ( -2.796473189345805913E-16, -40.43301269999997061, -98.84999999890752065 ) ) ;
#4220=ORIENTED_EDGE ( 'NONE', *, *, #4323, .T. ) ;
#4227=CARTESIAN_POINT ( 'NONE',  ( 4.566987300000000083, -46.89170807884564596, -99.89999999890751781 ) ) ;
#4228=CARTESIAN_POINT ( 'NONE',  ( -2.071067811865475505, -49.99999999999996447, -100.3499999978150754 ) ) ;
#4230=CARTESIAN_POINT ( 'NONE',  ( -1.891708078845683039, -40.43301269999998482, -98.59999999890754907 ) ) ;
#4235=CARTESIAN_POINT ( 'NONE',  ( -4.999999999999997335, -47.07106781186546129, -95.75000000000000000 ) ) ;
#4237=CARTESIAN_POINT ( 'NONE',  ( -4.566987299999998307, -43.10829192115428299, -96.89999999890751781 ) ) ;
#4247=CARTESIAN_POINT ( 'NONE',  ( 2.071067811865477282, -49.99999999999997158, -97.95000000000000284 ) ) ;
#4248=CARTESIAN_POINT ( 'NONE',  ( 3.535533905932737309, -48.53553390593270933, -99.39999999781504414 ) ) ;
#4250=SURFACE_STYLE_USAGE ( .BOTH. , #8183 ) ;
#4258=CARTESIAN_POINT ( 'NONE',  ( 3.229347689422839895, -41.77065231057713390, -96.34999999890753486 ) ) ;
#4262=CARTESIAN_POINT ( 'NONE',  ( 4.566987299999998307, -44.99999999999997158, -96.64999999890753202 ) ) ;
#4273=CARTESIAN_POINT ( 'NONE',  ( 3.535533905932736420, -41.46446609406723383, -99.99999999781503845 ) ) ;
#4275=CARTESIAN_POINT ( 'NONE',  ( 8.389419568037416259E-16, -49.56698729999997255, -99.84999999890753486 ) ) ;
#4280=CARTESIAN_POINT ( 'NONE',  ( -4.999999999999997335, -47.07106781186546129, -98.94300000002183992 ) ) ;
#4289=ADVANCED_FACE ( 'NONE', ( #5753 ), #8452, .T. ) ;
#4290=CARTESIAN_POINT ( 'NONE',  ( -4.999999999999997335, -47.07106781186546129, -98.15000000000000568 ) ) ;
#4299=CARTESIAN_POINT ( 'NONE',  ( -1.891708078845683039, -40.43301269999998482, -97.79999999890752349 ) ) ;
#4300=CARTESIAN_POINT ( 'NONE',  ( -4.999999999999998224, -44.99999999999997158, -99.79999999999999716 ) ) ;
#4302=CARTESIAN_POINT ( 'NONE',  ( 8.389419568037416259E-16, -49.56698729999997255, -99.24999999890751212 ) ) ;
#4305=CARTESIAN_POINT ( 'NONE',  ( -4.566987299999998307, -43.10829192115428299, -96.29999999890752349 ) ) ;
#4315=CARTESIAN_POINT ( 'NONE',  ( -5.000000000000007994, -42.92893218813450318, -98.14999999781504414 ) ) ;
#4316=CARTESIAN_POINT ( 'NONE',  ( 3.535533905932737309, -48.53553390593270933, -99.39999999781504414 ) ) ;
#4319=CARTESIAN_POINT ( 'NONE',  ( -1.891708078845683483, -49.56698729999997255, -98.29999999890752349 ) ) ;
#4323=EDGE_CURVE ( 'NONE', #6099, #6319, #4674, .T. ) ;
#4325=CARTESIAN_POINT ( 'NONE',  ( -3.061616997868382155E-16, -39.99999999999997158, -95.20000000000000284 ) ) ;
#4328=CARTESIAN_POINT ( 'NONE',  ( -2.071067811865475061, -39.99999999999997158, -97.44999999781505551 ) ) ;
#4331=CARTESIAN_POINT ( 'NONE',  ( -2.071067811865475061, -39.99999999999997158, -100.6499999978150441 ) ) ;
#4346=( BOUNDED_CURVE ( )  B_SPLINE_CURVE ( 2, ( #6929, #4825, #1553, #4247, #1468, #2273, #7634, #4290, #1424 ),
 .UNSPECIFIED., .F., .T. ) 
 B_SPLINE_CURVE_WITH_KNOTS ( ( 3, 2, 2, 2, 3 ),
 ( 0.5000000000000000000, 0.5178571428571429047, 0.5357142857142856984, 0.5535714285714286031, 0.5714285714285713969 ),
 .UNSPECIFIED. ) 
 CURVE ( )  GEOMETRIC_REPRESENTATION_ITEM ( )  RATIONAL_B_SPLINE_CURVE ( ( 1.000000000000000000, 0.9238795325112867385, 1.000000000000000000, 0.9238795325112867385, 1.000000000000000000, 0.9238795325112867385, 1.000000000000000000, 0.9238795325112867385, 1.000000000000000000 ) ) 
 REPRESENTATION_ITEM ( '' )  );
#4347=CARTESIAN_POINT ( 'NONE',  ( 4.566987300000000083, -46.89170807884564596, -99.69999999890752918 ) ) ;
#4350=CARTESIAN_POINT ( 'NONE',  ( -4.566987299999997418, -46.89170807884566727, -97.79999999890752349 ) ) ;
#4352=CARTESIAN_POINT ( 'NONE',  ( -4.566987299999998307, -44.99999999999997158, -97.04999999890752349 ) ) ;
#4353=CARTESIAN_POINT ( 'NONE',  ( -2.796473189345805913E-16, -40.43301269999997061, -100.4499999989075292 ) ) ;
#4361=CARTESIAN_POINT ( 'NONE',  ( 2.071067811865474173, -39.99999999999997158, -98.34999999781506119 ) ) ;
#4364=CARTESIAN_POINT ( 'NONE',  ( -4.999999999999998224, -44.99999999999997158, -96.60000000000000853 ) ) ;
#4370=CARTESIAN_POINT ( 'NONE',  ( 2.071067811865474173, -39.99999999999997158, -97.54999999781504982 ) ) ;
#4376=CARTESIAN_POINT ( 'NONE',  ( 2.071067811865477282, -49.99999999999997158, -97.04999999781504982 ) ) ;
#4384=ORIENTED_EDGE ( 'NONE', *, *, #1630, .T. ) ;
#4389=CARTESIAN_POINT ( 'NONE',  ( -3.229347689422839451, -48.22934768942280925, -99.14999999890753202 ) ) ;
#4394=CARTESIAN_POINT ( 'NONE',  ( -4.566987299999998307, -43.10829192115428299, -95.49999999890754054 ) ) ;
#4402=CARTESIAN_POINT ( 'NONE',  ( -2.071067811865475061, -39.99999999999997158, -96.64999999781505835 ) ) ;
#4404=CARTESIAN_POINT ( 'NONE',  ( -3.535533905932735532, -48.53553390593270933, -95.70000000000000284 ) ) ;
#4406=CARTESIAN_POINT ( 'NONE',  ( -4.999999999999998224, -44.99999999999997158, -95.00000000000000000 ) ) ;
#4413=CARTESIAN_POINT ( 'NONE',  ( 2.071067811865474173, -39.99999999999997158, -98.44999999999998863 ) ) ;
#4415=CARTESIAN_POINT ( 'NONE',  ( 9.184850993605145972E-16, -49.99999999999997158, -97.89999999781504414 ) ) ;
#4432=CARTESIAN_POINT ( 'NONE',  ( 1.891708078845685481, -49.56698729999997255, -98.99999999890752633 ) ) ;
#4435=CARTESIAN_POINT ( 'NONE',  ( -4.566987299999998307, -44.99999999999997158, -99.44999999890752918 ) ) ;
#4437=CARTESIAN_POINT ( 'NONE',  ( 4.566987299999998307, -43.10829192115428299, -97.39999999890751781 ) ) ;
#4449=CARTESIAN_POINT ( 'NONE',  ( -3.535533905932735532, -48.53553390593270933, -96.50000000000000000 ) ) ;
#4450=EDGE_LOOP ( 'NONE', ( #5563, #7962, #3091 ) ) ;
#4454=CARTESIAN_POINT ( 'NONE',  ( -4.999999999999997335, -47.07106781186546129, -98.15000000000000568 ) ) ;
#4455=CARTESIAN_POINT ( 'NONE',  ( 5.000000000000000000, -47.07106781186545419, -97.74999999781503845 ) ) ;
#4456=CARTESIAN_POINT ( 'NONE',  ( -4.135692067460690069, -42.17523997218626874, -100.0007971519677881 ) ) ;
#4458=CARTESIAN_POINT ( 'NONE',  ( 0.000000000000000000, -44.99999999999997158, -95.00000000000000000 ) ) ;
#4466=ORIENTED_EDGE ( 'NONE', *, *, #1671, .T. ) ;
#4470=CARTESIAN_POINT ( 'NONE',  ( 1.891708078845682595, -40.43301269999998482, -98.69999999890752918 ) ) ;
#4476=CARTESIAN_POINT ( 'NONE',  ( -2.796473189345805913E-16, -40.43301269999997061, -95.64999999890753202 ) ) ;
#4479=LINE ( 'NONE', #8456, #5952 ) ;
#4484=ADVANCED_FACE ( 'NONE', ( #2759 ), #6752, .T. ) ;
#4485=CARTESIAN_POINT ( 'NONE',  ( -4.999999999999998224, -44.99999999999997158, -95.69999999781504130 ) ) ;
#4487=CARTESIAN_POINT ( 'NONE',  ( -4.999999999999994671, -47.07106781186545419, -95.75000000000000000 ) ) ;
#4489=CARTESIAN_POINT ( 'NONE',  ( -3.061616997868382155E-16, -39.99999999999997158, -96.79999999999999716 ) ) ;
#4493=ORIENTED_EDGE ( 'NONE', *, *, #4779, .T. ) ;
#4494=CARTESIAN_POINT ( 'NONE',  ( -4.999999999999998224, -44.99999999999997158, -98.19999999999998863 ) ) ;
#4498=CARTESIAN_POINT ( 'NONE',  ( 0.000000000000000000, -44.99999999999997158, -95.00000000000000000 ) ) ;
#4499=CARTESIAN_POINT ( 'NONE',  ( 9.184850993605145972E-16, -49.99999999999997158, -97.09999999781504698 ) ) ;
#4510=CARTESIAN_POINT ( 'NONE',  ( 2.071067811865474173, -39.99999999999997158, -96.04999999999999716 ) ) ;
#4515=CARTESIAN_POINT ( 'NONE',  ( -2.796473189345805913E-16, -40.43301269999997061, -99.64999999890751781 ) ) ;
#4517=CARTESIAN_POINT ( 'NONE',  ( 4.566987299999998307, -43.10829192115428299, -95.59999999890754907 ) ) ;
#4526=ORIENTED_EDGE ( 'NONE', *, *, #130, .F. ) ;
#4530=PLANE ( 'NONE',  #5232 ) ;
#4533=CARTESIAN_POINT ( 'NONE',  ( 4.999999999999998224, -42.92893218813448897, -97.75000000000001421 ) ) ;
#4538=CARTESIAN_POINT ( 'NONE',  ( -3.535533905932735532, -48.53553390593270933, -98.90000000000000568 ) ) ;
#4544=CARTESIAN_POINT ( 'NONE',  ( 5.000000000000000000, -47.07106781186545419, -96.94999999781504130 ) ) ;
#4550=VECTOR ( 'NONE', #5097, 1000.000000000000000 ) ;
#4557=LINE ( 'NONE', #3287, #6147 ) ;
#4563=CARTESIAN_POINT ( 'NONE',  ( 1.891708078845682595, -40.43301269999998482, -98.89999999890751781 ) ) ;
#4565=ORIENTED_EDGE ( 'NONE', *, *, #7287, .F. ) ;
#4570=ORIENTED_EDGE ( 'NONE', *, *, #7226, .T. ) ;
#4577=CARTESIAN_POINT ( 'NONE',  ( -2.796473189345805913E-16, -40.43301269999997061, -100.4499999989075292 ) ) ;
#4582=CARTESIAN_POINT ( 'NONE',  ( -4.999999999999997335, -47.07106781186546129, -97.35000000000000853 ) ) ;
#4584=CARTESIAN_POINT ( 'NONE',  ( 4.566987300000000083, -46.89170807884565306, -98.09999999890752065 ) ) ;
#4589=CARTESIAN_POINT ( 'NONE',  ( 3.535533905932736420, -41.46446609406723383, -96.89300000002185698 ) ) ;
#4595=CARTESIAN_POINT ( 'NONE',  ( -4.999999999999998224, -44.99999999999997158, -99.79999999999999716 ) ) ;
#4596=AXIS2_PLACEMENT_3D ( 'NONE', #1482, #6249, #6946 ) ;
#4605=CARTESIAN_POINT ( 'NONE',  ( -4.999999999999998224, -44.99999999999997158, -99.79999999999999716 ) ) ;
#4606=CARTESIAN_POINT ( 'NONE',  ( -2.796473189345805913E-16, -40.43301269999997061, -98.84999999890752065 ) ) ;
#4617=CARTESIAN_POINT ( 'NONE',  ( 3.535533905932737309, -48.53553390593270933, -100.1999999978150555 ) ) ;
#4619=CARTESIAN_POINT ( 'NONE',  ( 3.535533905932736420, -41.46446609406723383, -98.50000000000000000 ) ) ;
#4620=VERTEX_POINT ( 'NONE', #3593 ) ;
#4622=( BOUNDED_CURVE ( )  B_SPLINE_CURVE ( 2, ( #1436, #3476, #6896, #3559, #6157, #6282, #6242, #2943, #241, #114, #4172, #2813, #5572, #4790, #1563, #1477, #7558, #201, #5484, #4963, #6984, #2904, #4258, #8193, #3643, #8237, #2282, #6197, #4131, #2151, #6941, #8320, #4213, #4838, #6853, #4920, #7600, #3601, #8364, #817, #3518, #5618, #160, #1520, #2195, #2856, #7474, #7646, #1610, #5531, #6323, #4299, #948, #286, #4880, #2988, #5662, #3853, #8486, #442, #7737, #1789, #3033, #1158, #5750, #8525, #3728, #7695, #5705, #4470, #5835, #6533, #2451, #8408, #5132, #4432, #1077, #987, #4389, #2491, #2328, #365, #482, #7779, #3074, #1656, #7824, #3197, #7115, #4347, #7156, #3771, #5880, #5172, #2373, #6491, #5006, #7027, #1749, #1116, #3686 ),
 .UNSPECIFIED., .F., .T. ) 
 B_SPLINE_CURVE_WITH_KNOTS ( ( 3, 2, 2, 2, 2, 2, 2, 2, 2, 2, 2, 2, 2, 2, 2, 2, 2, 2, 2, 2, 2, 2, 2, 2, 2, 2, 2, 2, 2, 2, 2, 2, 2, 2, 2, 2, 2, 2, 2, 2, 2, 2, 2, 2, 2, 2, 2, 2, 2, 2, 3 ),
 ( 0.000000000000000000, 0.01785714285714285615, 0.03571428571428571230, 0.05357142857142856845, 0.07142857142857142461, 0.08928571428571428770, 0.1071428571428571369, 0.1250000000000000000, 0.1428571428571428492, 0.1607142857142857262, 0.1785714285714285754, 0.1964285714285714246, 0.2142857142857142738, 0.2321428571428571508, 0.2500000000000000000, 0.2678571428571428492, 0.2857142857142856984, 0.3035714285714285476, 0.3214285714285714524, 0.3392857142857143016, 0.3571428571428571508, 0.3750000000000000000, 0.3928571428571428492, 0.4107142857142856984, 0.4285714285714285476, 0.4464285714285714524, 0.4642857142857143016, 0.4821428571428571508, 0.5000000000000000000, 0.5178571428571429047, 0.5357142857142856984, 0.5535714285714286031, 0.5714285714285713969, 0.5892857142857143016, 0.6071428571428570953, 0.6250000000000000000, 0.6428571428571429047, 0.6607142857142856984, 0.6785714285714286031, 0.6964285714285715079, 0.7142857142857143016, 0.7321428571428570953, 0.7500000000000000000, 0.7678571428571429047, 0.7857142857142856984, 0.8035714285714286031, 0.8214285714285713969, 0.8392857142857143016, 0.8571428571428570953, 0.8750000000000000000, 0.8928571428571429047 ),
 .UNSPECIFIED. ) 
 CURVE ( )  GEOMETRIC_REPRESENTATION_ITEM ( )  RATIONAL_B_SPLINE_CURVE ( ( 1.000000000000000000, 0.9238795325112867385, 1.000000000000000000, 0.9238795325112867385, 1.000000000000000000, 0.9238795325112867385, 1.000000000000000000, 0.9238795325112867385, 1.000000000000000000, 0.9238795325112867385, 1.000000000000000000, 0.9238795325112867385, 1.000000000000000000, 0.9238795325112867385, 1.000000000000000000, 0.9238795325112867385, 1.000000000000000000, 0.9238795325112867385, 1.000000000000000000, 0.9238795325112867385, 1.000000000000000000, 0.9238795325112867385, 1.000000000000000000, 0.9238795325112867385, 1.000000000000000000, 0.9238795325112867385, 1.000000000000000000, 0.9238795325112867385, 1.000000000000000000, 0.9238795325112867385, 1.000000000000000000, 0.9238795325112867385, 1.000000000000000000, 0.9238795325112867385, 1.000000000000000000, 0.9238795325112867385, 1.000000000000000000, 0.9238795325112867385, 1.000000000000000000, 0.9238795325112867385, 1.000000000000000000, 0.9238795325112867385, 1.000000000000000000, 0.9238795325112867385, 1.000000000000000000, 0.9238795325112867385, 1.000000000000000000, 0.9238795325112867385, 1.000000000000000000, 0.9238795325112867385, 1.000000000000000000, 0.9238795325112867385, 1.000000000000000000, 0.9238795325112867385, 1.000000000000000000, 0.9238795325112867385, 1.000000000000000000, 0.9238795325112867385, 1.000000000000000000, 0.9238795325112867385, 1.000000000000000000, 0.9238795325112867385, 1.000000000000000000, 0.9238795325112867385, 1.000000000000000000, 0.9238795325112867385, 1.000000000000000000, 0.9238795325112867385, 1.000000000000000000, 0.9238795325112867385, 1.000000000000000000, 0.9238795325112867385, 1.000000000000000000, 0.9238795325112867385, 1.000000000000000000, 0.9238795325112867385, 1.000000000000000000, 0.9238795325112867385, 1.000000000000000000, 0.9238795325112867385, 1.000000000000000000, 0.9238795325112867385, 1.000000000000000000, 0.9238795325112867385, 1.000000000000000000, 0.9238795325112867385, 1.000000000000000000, 0.9238795325112867385, 1.000000000000000000, 0.9238795325112867385, 1.000000000000000000, 0.9238795325112867385, 1.000000000000000000, 0.9238795325112867385, 1.000000000000000000, 0.9238795325112867385, 1.000000000000000000, 0.9238795325112867385, 1.000000000000000000, 0.9238795325112867385, 1.000000000000000000 ) ) 
 REPRESENTATION_ITEM ( '' )  );
#4625=CARTESIAN_POINT ( 'NONE',  ( -2.071067811865475061, -39.99999999999997158, -95.84999999781503277 ) ) ;
#4627=CARTESIAN_POINT ( 'NONE',  ( -3.229347689422840784, -41.77065231057713390, -99.34999999890753486 ) ) ;
#4630=CARTESIAN_POINT ( 'NONE',  ( -3.061616997868382155E-16, -39.99999999999997158, -97.59300000002185982 ) ) ;
#4636=CARTESIAN_POINT ( 'NONE',  ( 7.499999999999999112, -44.99999999999997158, -105.0000000000000142 ) ) ;
#4640=DIRECTION ( 'NONE',  ( 0.000000000000000000, 0.000000000000000000, 1.000000000000000000 ) ) ;
#4641=LINE ( 'NONE', #2668, #8130 ) ;
#4646=CARTESIAN_POINT ( 'NONE',  ( 3.229347689422841228, -48.22934768942280925, -99.94999999890752918 ) ) ;
#4658=CARTESIAN_POINT ( 'NONE',  ( 3.535533905932736420, -41.46446609406723383, -99.99999999781503845 ) ) ;
#4659=CARTESIAN_POINT ( 'NONE',  ( -2.071067811865475061, -39.99999999999997158, -95.14999999999999147 ) ) ;
#4660=CARTESIAN_POINT ( 'NONE',  ( 4.999999999999998224, -42.92893218813448897, -98.54999999999999716 ) ) ;
#4667=CARTESIAN_POINT ( 'NONE',  ( 3.229347689422841228, -48.22934768942280925, -99.14999999890751781 ) ) ;
#4668=EDGE_CURVE ( 'NONE', #4620, #799, #4346, .T. ) ;
#4669=CARTESIAN_POINT ( 'NONE',  ( -2.071067811865475505, -49.99999999999996447, -99.64999999999999147 ) ) ;
#4671=CARTESIAN_POINT ( 'NONE',  ( -4.566987299999998307, -44.99999999999997158, -97.64999999890753202 ) ) ;
#4672=SURFACE_STYLE_FILL_AREA ( #4148 ) ;
#4674=( BOUNDED_CURVE ( )  B_SPLINE_CURVE ( 2, ( #3202, #5885, #6097, #6667, #5925, #1331, #5966, #56, #622 ),
 .UNSPECIFIED., .F., .T. ) 
 B_SPLINE_CURVE_WITH_KNOTS ( ( 3, 2, 2, 2, 3 ),
 ( 0.5714285714285713969, 0.5892857142857143016, 0.6071428571428570953, 0.6250000000000000000, 0.6428571428571429047 ),
 .UNSPECIFIED. ) 
 CURVE ( )  GEOMETRIC_REPRESENTATION_ITEM ( )  RATIONAL_B_SPLINE_CURVE ( ( 1.000000000000000000, 0.9238795325112867385, 1.000000000000000000, 0.9238795325112867385, 1.000000000000000000, 0.9238795325112867385, 1.000000000000000000, 0.9238795325112867385, 1.000000000000000000 ) ) 
 REPRESENTATION_ITEM ( '' )  );
#4676=CARTESIAN_POINT ( 'NONE',  ( 4.999999999999998224, -42.92893218813448897, -96.14300000002184277 ) ) ;
#4677=CIRCLE ( 'NONE', #5806, 7.499999999999999112 ) ;
#4684=CARTESIAN_POINT ( 'NONE',  ( 4.999999999999998224, -44.99999999999997158, -99.40000000000000568 ) ) ;
#4696=CARTESIAN_POINT ( 'NONE',  ( -4.566987299999998307, -43.10829192115428299, -96.09999999890752065 ) ) ;
#4705=EDGE_CURVE ( 'NONE', #2692, #7480, #423, .T. ) ;
#4708=CARTESIAN_POINT ( 'NONE',  ( -3.535533905932736864, -41.46446609406723383, -98.19999999781505551 ) ) ;
#4710=CARTESIAN_POINT ( 'NONE',  ( 3.535533905932737309, -48.53553390593270933, -98.70000000000000284 ) ) ;
#4716=CARTESIAN_POINT ( 'NONE',  ( 3.229347689422839895, -41.77065231057713390, -96.54999999890752349 ) ) ;
#4717=CARTESIAN_POINT ( 'NONE',  ( -3.535533905932736864, -41.46446609406723383, -97.39999999781504414 ) ) ;
#4719=CARTESIAN_POINT ( 'NONE',  ( 4.566987299999998307, -43.10829192115428299, -98.79999999890753770 ) ) ;
#4722=CARTESIAN_POINT ( 'NONE',  ( 3.535533905932736420, -41.46446609406723383, -96.09300000002185982 ) ) ;
#4723=VECTOR ( 'NONE', #6997, 1000.000000000000000 ) ;
#4726=CARTESIAN_POINT ( 'NONE',  ( -4.999999999999998224, -44.99999999999997158, -95.69999999781504130 ) ) ;
#4733=CARTESIAN_POINT ( 'NONE',  ( 4.999999999999994671, -42.92893218813449607, -96.95000000000000284 ) ) ;
#4734=CARTESIAN_POINT ( 'NONE',  ( -4.999999999999998224, -44.99999999999997158, -95.00000000000000000 ) ) ;
#4739=CARTESIAN_POINT ( 'NONE',  ( 8.389419568037416259E-16, -49.56698729999997255, -96.64999999890753202 ) ) ;
#4749=CARTESIAN_POINT ( 'NONE',  ( 9.184850993605145972E-16, -49.99999999999997158, -98.69999999781505551 ) ) ;
#4750=CARTESIAN_POINT ( 'NONE',  ( 4.999999999999998224, -44.99999999999997158, -96.20000000000000284 ) ) ;
#4760=CARTESIAN_POINT ( 'NONE',  ( -4.566987299999998307, -44.99999999999997158, -97.04999999890752349 ) ) ;
#4761=CARTESIAN_POINT ( 'NONE',  ( 2.071067811865477282, -49.99999999999996447, -97.84999999781504698 ) ) ;
#4764=CARTESIAN_POINT ( 'NONE',  ( 1.891708078845685481, -49.56698729999997255, -98.99999999890752633 ) ) ;
#4765=FACE_OUTER_BOUND ( 'NONE', #4450, .T. ) ;
#4767=CARTESIAN_POINT ( 'NONE',  ( 9.184850993605145972E-16, -49.99999999999997158, -96.39300000002185698 ) ) ;
#4771=CARTESIAN_POINT ( 'NONE',  ( 4.999999999999998224, -44.99999999999997158, -96.09999999781504698 ) ) ;
#4773=CARTESIAN_POINT ( 'NONE',  ( -2.071067811865475505, -49.99999999999997158, -99.65000000000000568 ) ) ;
#4779=EDGE_CURVE ( 'NONE', #196, #2012, #8181, .T. ) ;
#4782=SURFACE_STYLE_FILL_AREA ( #4827 ) ;
#4790=CARTESIAN_POINT ( 'NONE',  ( -1.891708078845683705, -49.56698729999997255, -95.89999999890753202 ) ) ;
#4791=CARTESIAN_POINT ( 'NONE',  ( -2.796473189345805913E-16, -40.43301269999997061, -100.2499999989075263 ) ) ;
#4794=CARTESIAN_POINT ( 'NONE',  ( 8.389419568037416259E-16, -49.56698729999997255, -96.04999999890752349 ) ) ;
#4797=EDGE_CURVE ( 'NONE', #6586, #7878, #5341, .T. ) ;
#4803=CARTESIAN_POINT ( 'NONE',  ( -1.891708078845683039, -40.43301269999998482, -97.19999999890751496 ) ) ;
#4804=CARTESIAN_POINT ( 'NONE',  ( -4.999999999999998224, -46.91341716182541433, -95.65380602118948161 ) ) ;
#4807=CARTESIAN_POINT ( 'NONE',  ( 1.891708078845682595, -40.43301269999998482, -97.09999999890753486 ) ) ;
#4811=CARTESIAN_POINT ( 'NONE',  ( 4.999999999999998224, -44.99999999999997158, -98.59300000002185982 ) ) ;
#4813=CARTESIAN_POINT ( 'NONE',  ( -3.229347689422839451, -48.22934768942280925, -97.54999999890752349 ) ) ;
#4822=DIRECTION ( 'NONE',  ( -0.000000000000000000, -0.000000000000000000, -1.000000000000000000 ) ) ;
#4825=CARTESIAN_POINT ( 'NONE',  ( 5.000000000000000000, -47.07106781186545419, -97.85000000000003695 ) ) ;
#4827=FILL_AREA_STYLE ('',( #2099 ) ) ;
#4838=CARTESIAN_POINT ( 'NONE',  ( -4.566987299999998307, -43.10829192115428299, -96.89999999890753202 ) ) ;
#4841=CARTESIAN_POINT ( 'NONE',  ( -1.891708078845683039, -40.43301269999998482, -96.39999999890753202 ) ) ;
#4852=CARTESIAN_POINT ( 'NONE',  ( -3.229347689422839451, -48.22934768942280925, -97.74999999890751212 ) ) ;
#4855=CARTESIAN_POINT ( 'NONE',  ( -4.566987299999998307, -44.99999999999997158, -99.24999999890752633 ) ) ;
#4858=CARTESIAN_POINT ( 'NONE',  ( -2.071067811865475061, -39.99999999999997158, -99.94300000002185413 ) ) ;
#4872=CARTESIAN_POINT ( 'NONE',  ( -4.783493649999997821, -44.99999999999997158, -95.57499999836127813 ) ) ;
#4880=CARTESIAN_POINT ( 'NONE',  ( 3.229347689422839895, -41.77065231057713390, -97.94999999890751496 ) ) ;
#4883=CARTESIAN_POINT ( 'NONE',  ( 1.891708078845685481, -49.56698729999997255, -96.79999999890753770 ) ) ;
#4894=CARTESIAN_POINT ( 'NONE',  ( 4.566987299999998307, -43.10829192115428299, -99.79999999890752349 ) ) ;
#4895=CARTESIAN_POINT ( 'NONE',  ( 4.999999999999998224, -44.99999999999997158, -100.0999999978150470 ) ) ;
#4897=CARTESIAN_POINT ( 'NONE',  ( -4.566987299999998307, -43.10829192115428299, -99.29999999890752349 ) ) ;
#4901=CARTESIAN_POINT ( 'NONE',  ( -2.071067811865475061, -39.99999999999997158, -95.95000000000003126 ) ) ;
#4902=CARTESIAN_POINT ( 'NONE',  ( -3.229347689422839451, -48.22934768942280925, -96.74999999890752633 ) ) ;
#4906=( BOUNDED_CURVE ( )  B_SPLINE_CURVE ( 2, ( #4750, #4046, #27, #2728, #3216, #5899, #640, #1180, #6592 ),
 .UNSPECIFIED., .F., .T. ) 
 B_SPLINE_CURVE_WITH_KNOTS ( ( 3, 2, 2, 2, 3 ),
 ( 0.2142857142857142738, 0.2321428571428571508, 0.2499999999999999722, 0.2678571428571427937, 0.2857142857142856429 ),
 .UNSPECIFIED. ) 
 CURVE ( )  GEOMETRIC_REPRESENTATION_ITEM ( )  RATIONAL_B_SPLINE_CURVE ( ( 1.000000000000000000, 0.9238795325112867385, 1.000000000000000000, 0.9238795325112867385, 1.000000000000000000, 0.9238795325112867385, 1.000000000000000000, 0.9238795325112869605, 0.9999999999999997780 ) ) 
 REPRESENTATION_ITEM ( '' )  );
#4912=PRESENTATION_STYLE_ASSIGNMENT (( #4250 ) ) ;
#4920=CARTESIAN_POINT ( 'NONE',  ( -1.891708078845683039, -40.43301269999998482, -96.99999999890752633 ) ) ;
#4923=CARTESIAN_POINT ( 'NONE',  ( -1.891708078845683483, -49.56698729999997255, -97.69999999890751496 ) ) ;
#4929=ORIENTED_EDGE ( 'NONE', *, *, #130, .T. ) ;
#4931=DIRECTION ( 'NONE',  ( -0.000000000000000000, -0.000000000000000000, -1.000000000000000000 ) ) ;
#4933=CARTESIAN_POINT ( 'NONE',  ( -3.535533905932736864, -41.46446609406723383, -99.79999999781504982 ) ) ;
#4934=CARTESIAN_POINT ( 'NONE',  ( -2.071067811865475505, -49.99999999999997158, -97.94999999781505551 ) ) ;
#4935=CARTESIAN_POINT ( 'NONE',  ( -2.796473189345805913E-16, -40.43301269999997061, -99.44999999890752918 ) ) ;
#4942=CARTESIAN_POINT ( 'NONE',  ( 3.535533905932737309, -48.53553390593270933, -98.69300000002183992 ) ) ;
#4944=CARTESIAN_POINT ( 'NONE',  ( 4.999999999999998224, -44.99999999999997158, -96.09999999781504698 ) ) ;
#4960=ADVANCED_FACE ( 'NONE', ( #5125 ), #7816, .T. ) ;
#4963=CARTESIAN_POINT ( 'NONE',  ( -1.891708078845683039, -40.43301269999998482, -96.19999999890752918 ) ) ;
#4967=CARTESIAN_POINT ( 'NONE',  ( 4.566987299999998307, -43.10829192115428299, -96.59999999890753486 ) ) ;
#4969=CARTESIAN_POINT ( 'NONE',  ( 4.566987300000000083, -46.89170807884565306, -98.29999999890752349 ) ) ;
#4980=CARTESIAN_POINT ( 'NONE',  ( 3.535533905932736420, -41.46446609406723383, -98.39999999781504414 ) ) ;
#4981=CARTESIAN_POINT ( 'NONE',  ( 5.000000000000000000, -47.07106781186545419, -99.34999999781506119 ) ) ;
#4983=CARTESIAN_POINT ( 'NONE',  ( 4.566987299999998307, -43.10829192115428299, -97.19999999890752918 ) ) ;
#4987=CARTESIAN_POINT ( 'NONE',  ( 3.535533905932737309, -48.53553390593270933, -99.49300000002185129 ) ) ;
#4994=CARTESIAN_POINT ( 'NONE',  ( 3.229347689422841228, -48.22934768942280925, -95.94999999890751496 ) ) ;
#5005=ADVANCED_FACE ( 'NONE', ( #3720 ), #3801, .T. ) ;
#5006=CARTESIAN_POINT ( 'NONE',  ( -4.566987299999998307, -44.99999999999997158, -100.0499999989075235 ) ) ;
#5010=CARTESIAN_POINT ( 'NONE',  ( -4.566987299999997418, -46.89170807884566727, -96.19999999890751496 ) ) ;
#5012=AXIS2_PLACEMENT_3D ( 'NONE', #8307, #758, #2181 ) ;
#5013=CARTESIAN_POINT ( 'NONE',  ( 1.891708078845682595, -40.43301269999998482, -97.29999999890750928 ) ) ;
#5020=DIRECTION ( 'NONE',  ( -1.000000000000000000, 0.000000000000000000, 0.000000000000000000 ) ) ;
#5021=CARTESIAN_POINT ( 'NONE',  ( -1.891708078845683039, -40.43301269999998482, -100.3999999989075178 ) ) ;
#5022=CARTESIAN_POINT ( 'NONE',  ( 2.071067811865477282, -49.99999999999996447, -99.44999999781505551 ) ) ;
#5024=CARTESIAN_POINT ( 'NONE',  ( 5.000000000000000000, -47.07106781186545419, -97.85000000000002274 ) ) ;
#5031=CARTESIAN_POINT ( 'NONE',  ( 3.535533905932737309, -48.53553390593270933, -96.19999999781504130 ) ) ;
#5033=CARTESIAN_POINT ( 'NONE',  ( -4.999999999999998224, -44.99999999999997158, -98.89999999781504414 ) ) ;
#5036=DIRECTION ( 'NONE',  ( 0.000000000000000000, 0.000000000000000000, 1.000000000000000000 ) ) ;
#5037=CARTESIAN_POINT ( 'NONE',  ( 2.071067811865474173, -39.99999999999997158, -98.45000000000000284 ) ) ;
#5053=CARTESIAN_POINT ( 'NONE',  ( 3.229347689422841228, -48.22934768942280925, -97.54999999890752349 ) ) ;
#5060=CARTESIAN_POINT ( 'NONE',  ( -4.999999999999998224, -44.99999999999997158, -96.49999999781503845 ) ) ;
#5063=CARTESIAN_POINT ( 'NONE',  ( -2.071067811865475061, -39.99999999999997158, -97.44999999781504130 ) ) ;
#5065=CARTESIAN_POINT ( 'NONE',  ( 9.184850993605145972E-16, -49.99999999999997158, -97.19999999999998863 ) ) ;
#5066=B_SPLINE_CURVE_WITH_KNOTS ( 'NONE', 1,
 ( #8151, #3388 ),
 .UNSPECIFIED., .F., .F.,
 ( 2, 2 ),
 ( 0.000000000000000000, 1.000000000000000000 ),
 .UNSPECIFIED. ) ;
#5070=CARTESIAN_POINT ( 'NONE',  ( 3.535533905932737309, -48.53553390593270933, -97.90000000000000568 ) ) ;
#5071=CARTESIAN_POINT ( 'NONE',  ( -4.999999999999998224, -44.99999999999997158, -95.69999999781504130 ) ) ;
#5077=CARTESIAN_POINT ( 'NONE',  ( -2.071067811865475061, -39.99999999999997158, -99.84999999781504698 ) ) ;
#5093=CARTESIAN_POINT ( 'NONE',  ( -4.566987299999998307, -43.10829192115428299, -99.49999999890754054 ) ) ;
#5095=CARTESIAN_POINT ( 'NONE',  ( -1.891708078845683039, -40.43301269999998482, -96.39999999890753202 ) ) ;
#5096=ORIENTED_EDGE ( 'NONE', *, *, #515, .T. ) ;
#5097=DIRECTION ( 'NONE',  ( -0.000000000000000000, -0.000000000000000000, -1.000000000000000000 ) ) ;
#5105=CARTESIAN_POINT ( 'NONE',  ( 0.000000000000000000, -44.99999999999997158, -95.00000000000000000 ) ) ;
#5107=LINE ( 'NONE', #2550, #3273 ) ;
#5108=CARTESIAN_POINT ( 'NONE',  ( 9.184850993605145972E-16, -49.99999999999997158, -96.40000000000000568 ) ) ;
#5113=ORIENTED_EDGE ( 'NONE', *, *, #786, .F. ) ;
#5114=EDGE_CURVE ( 'NONE', #6251, #4620, #8243, .T. ) ;
#5115=CARTESIAN_POINT ( 'NONE',  ( 3.535533905932736420, -41.46446609406723383, -96.90000000000000568 ) ) ;
#5118=CARTESIAN_POINT ( 'NONE',  ( -4.270064113631143243, -47.61730482574012058, -99.99930497888919945 ) ) ;
#5120=FACE_OUTER_BOUND ( 'NONE', #2146, .T. ) ;
#5121=CARTESIAN_POINT ( 'NONE',  ( -3.535533905932735532, -48.53553390593270933, -97.19999999781504130 ) ) ;
#5125=FACE_OUTER_BOUND ( 'NONE', #8278, .T. ) ;
#5132=CARTESIAN_POINT ( 'NONE',  ( 3.229347689422841228, -48.22934768942280925, -98.94999999890752918 ) ) ;
#5137=CARTESIAN_POINT ( 'NONE',  ( 4.566987299999998307, -44.99999999999997158, -96.64999999890753202 ) ) ;
#5143=VERTEX_POINT ( 'NONE', #1011 ) ;
#5148=CARTESIAN_POINT ( 'NONE',  ( -5.000000000000002665, -47.07106781186544708, -97.34999999999999432 ) ) ;
#5151=CARTESIAN_POINT ( 'NONE',  ( 3.535533905932737309, -48.53553390593270933, -95.50000000000000000 ) ) ;
#5152=VERTEX_POINT ( 'NONE', #8562 ) ;
#5156=CARTESIAN_POINT ( 'NONE',  ( 9.184850993605145972E-16, -49.99999999999997158, -97.19999999999998863 ) ) ;
#5157=CARTESIAN_POINT ( 'NONE',  ( 0.04104470510518735960, -50.00775265013817972, -99.99997323207621491 ) ) ;
#5160=CARTESIAN_POINT ( 'NONE',  ( -4.999999999999998224, -46.91341716182541433, -94.94680602339629161 ) ) ;
#5172=CARTESIAN_POINT ( 'NONE',  ( -1.891708078845683705, -49.56698729999997255, -99.89999999890753202 ) ) ;
#5178=CARTESIAN_POINT ( 'NONE',  ( 1.891708078845685481, -49.56698729999997255, -95.79999999890752349 ) ) ;
#5189=CARTESIAN_POINT ( 'NONE',  ( -3.535533905932736864, -41.46446609406723383, -96.70000000000000284 ) ) ;
#5194=CARTESIAN_POINT ( 'NONE',  ( 4.999999999999998224, -44.99999999999997158, -97.00000000000000000 ) ) ;
#5195=CARTESIAN_POINT ( 'NONE',  ( 3.930156119229561540, -41.85908832164993498, -99.99888990999863836 ) ) ;
#5198=CARTESIAN_POINT ( 'NONE',  ( -2.071067811865475505, -49.99999999999997158, -97.14999999781504414 ) ) ;
#5215=CARTESIAN_POINT ( 'NONE',  ( -4.566987299999997418, -46.89170807884566727, -100.1999999989075150 ) ) ;
#5217=CARTESIAN_POINT ( 'NONE',  ( -3.229347689422840784, -41.77065231057713390, -100.3499999989075206 ) ) ;
#5219=DIRECTION ( 'NONE',  ( -0.000000000000000000, -0.000000000000000000, -1.000000000000000000 ) ) ;
#5225=CARTESIAN_POINT ( 'NONE',  ( -4.999999999999998224, -42.92893218813449607, -99.04999999999999716 ) ) ;
#5226=CARTESIAN_POINT ( 'NONE',  ( -4.999999999999997335, -47.07106781186546129, -96.44999999781505551 ) ) ;
#5232=AXIS2_PLACEMENT_3D ( 'NONE', #341, #1003, #7044 ) ;
#5236=CARTESIAN_POINT ( 'NONE',  ( -4.999999999999998224, -44.99999999999997158, -96.60000000000000853 ) ) ;
#5238=CARTESIAN_POINT ( 'NONE',  ( -1.891708078845683483, -49.56698729999997255, -97.49999999890754054 ) ) ;
#5240=CARTESIAN_POINT ( 'NONE',  ( 4.472107766621025604, -47.30873943526144387, -100.0006001545488203 ) ) ;
#5244=CARTESIAN_POINT ( 'NONE',  ( -2.071067811865475061, -39.99999999999997158, -97.54999999999998295 ) ) ;
#5257=CARTESIAN_POINT ( 'NONE',  ( -4.566987299999998307, -43.10829192115428299, -100.2999999989075093 ) ) ;
#5262=ORIENTED_EDGE ( 'NONE', *, *, #3105, .T. ) ;
#5267=CARTESIAN_POINT ( 'NONE',  ( -3.061616997868382155E-16, -39.99999999999997158, -98.29999999781504982 ) ) ;
#5269=CARTESIAN_POINT ( 'NONE',  ( 3.535533905932737309, -48.53553390593270933, -99.50000000000000000 ) ) ;
#5274=CARTESIAN_POINT ( 'NONE',  ( -3.061616997868382155E-16, -39.99999999999997158, -95.89999999781505835 ) ) ;
#5276=CARTESIAN_POINT ( 'NONE',  ( -4.566987299999997418, -46.89170807884566727, -98.39999999890753202 ) ) ;
#5277=CARTESIAN_POINT ( 'NONE',  ( 1.168677208981296678, -49.87010530342148940, -100.0006950213451233 ) ) ;
#5279=CARTESIAN_POINT ( 'NONE',  ( 4.999999999999998224, -44.99999999999997158, -97.79300000002184845 ) ) ;
#5297=CARTESIAN_POINT ( 'NONE',  ( -4.566987299999998307, -43.10829192115428299, -95.29999999890750928 ) ) ;
#5301=CARTESIAN_POINT ( 'NONE',  ( -4.999999999999997335, -47.07106781186546129, -98.95000000000000284 ) ) ;
#5312=CARTESIAN_POINT ( 'NONE',  ( 2.071067811865477282, -49.99999999999996447, -99.44999999781505551 ) ) ;
#5314=CARTESIAN_POINT ( 'NONE',  ( 2.071067811865477282, -49.99999999999996447, -98.75000000000001421 ) ) ;
#5319=VERTEX_POINT ( 'NONE', #1864 ) ;
#5320=CARTESIAN_POINT ( 'NONE',  ( 4.566987299999998307, -44.99999999999997158, -99.04999999890752349 ) ) ;
#5321=CARTESIAN_POINT ( 'NONE',  ( 4.999999999999998224, -44.99999999999997158, -99.40000000000000568 ) ) ;
#5323=CARTESIAN_POINT ( 'NONE',  ( 1.891708078845685481, -49.56698729999997255, -97.39999999890751781 ) ) ;
#5324=FILL_AREA_STYLE_COLOUR ( '', #6061 ) ;
#5327=CARTESIAN_POINT ( 'NONE',  ( 4.999999999999998224, -44.99999999999997158, -95.39300000002184277 ) ) ;
#5329=CARTESIAN_POINT ( 'NONE',  ( -4.999999999999994671, -42.92893218813449607, -97.45000000000000284 ) ) ;
#5331=ORIENTED_EDGE ( 'NONE', *, *, #5517, .T. ) ;
#5340=CARTESIAN_POINT ( 'NONE',  ( 8.389419568037416259E-16, -49.56698729999997255, -95.84999999890753486 ) ) ;
#5341=CIRCLE ( 'NONE', #1282, 7.499999999999999112 ) ;
#5352=CARTESIAN_POINT ( 'NONE',  ( 2.071067811865477282, -49.99999999999996447, -98.64999999781504414 ) ) ;
#5353=CARTESIAN_POINT ( 'NONE',  ( 3.535533905932736420, -41.46446609406723383, -95.29999999999999716 ) ) ;
#5362=CARTESIAN_POINT ( 'NONE',  ( -4.566987299999997418, -46.89170807884566017, -99.39999999890751781 ) ) ;
#5363=CARTESIAN_POINT ( 'NONE',  ( -3.535533905932736864, -41.46446609406723383, -96.59999999781504698 ) ) ;
#5365=CARTESIAN_POINT ( 'NONE',  ( -3.229347689422840784, -41.77065231057713390, -97.74999999890752633 ) ) ;
#5369=CARTESIAN_POINT ( 'NONE',  ( -2.071067811865475505, -49.99999999999996447, -98.04300000002186266 ) ) ;
#5383=CARTESIAN_POINT ( 'NONE',  ( -4.999999999999998224, -44.99999999999997158, -99.69999999781505551 ) ) ;
#5384=CARTESIAN_POINT ( 'NONE',  ( -1.891708078845683483, -49.56698729999997255, -96.69999999890755760 ) ) ;
#5397=CARTESIAN_POINT ( 'NONE',  ( -4.999999999999997335, -47.07106781186546129, -98.84999999781503277 ) ) ;
#5399=CARTESIAN_POINT ( 'NONE',  ( -3.061616997868382155E-16, -39.99999999999997158, -100.0000000000000000 ) ) ;
#5406=CARTESIAN_POINT ( 'NONE',  ( 4.566987299999998307, -43.10829192115428299, -97.39999999890753202 ) ) ;
#5407=CARTESIAN_POINT ( 'NONE',  ( 5.000000000000000000, -47.07106781186545419, -97.74999999781503845 ) ) ;
#5409=CARTESIAN_POINT ( 'NONE',  ( -1.891708078845683483, -49.56698729999997255, -99.09999999890753486 ) ) ;
#5410=DIRECTION ( 'NONE',  ( -1.000000000000000000, 0.000000000000000000, -0.000000000000000000 ) ) ;
#5413=CARTESIAN_POINT ( 'NONE',  ( 2.071067811865474173, -39.99999999999997158, -95.24300000002185129 ) ) ;
#5430=CARTESIAN_POINT ( 'NONE',  ( 4.999999999999998224, -44.99999999999997158, -99.29999999781504982 ) ) ;
#5440=CARTESIAN_POINT ( 'NONE',  ( -4.999999999999998224, -44.99999999999997158, -99.69999999781505551 ) ) ;
#5448=DIRECTION ( 'NONE',  ( -1.000000000000000000, 0.000000000000000000, 0.000000000000000000 ) ) ;
#5449=CARTESIAN_POINT ( 'NONE',  ( -2.796473189345805913E-16, -40.43301269999997061, -98.04999999890752349 ) ) ;
#5450=CARTESIAN_POINT ( 'NONE',  ( 4.999999999999998224, -44.99999999999997158, -96.09999999781504698 ) ) ;
#5453=CARTESIAN_POINT ( 'NONE',  ( 8.389419568037416259E-16, -49.56698729999997255, -97.44999999890751496 ) ) ;
#5458=CARTESIAN_POINT ( 'NONE',  ( 9.184850993605145972E-16, -49.99999999999997158, -95.59300000002185982 ) ) ;
#5462=EDGE_CURVE ( 'NONE', #2812, #6772, #2894, .T. ) ;
#5471=CARTESIAN_POINT ( 'NONE',  ( -7.654042494670954648E-16, -39.99999999999997158, -100.0000000000000000 ) ) ;
#5484=CARTESIAN_POINT ( 'NONE',  ( -3.229347689422840784, -41.77065231057713390, -96.14999999890753202 ) ) ;
#5488=CARTESIAN_POINT ( 'NONE',  ( 4.566987299999998307, -43.10829192115428299, -97.39999999890751781 ) ) ;
#5494=ORIENTED_EDGE ( 'NONE', *, *, #3230, .F. ) ;
#5496=CARTESIAN_POINT ( 'NONE',  ( -4.999999999999998224, -44.99999999999997158, -98.89999999781504414 ) ) ;
#5497=CARTESIAN_POINT ( 'NONE',  ( 3.229347689422839895, -41.77065231057713390, -98.14999999890751781 ) ) ;
#5498=CARTESIAN_POINT ( 'NONE',  ( -4.999999999999998224, -44.99999999999997158, -100.4999999978150385 ) ) ;
#5499=STYLED_ITEM ( 'NONE', ( #6693 ), #8634 ) ;
#5501=CARTESIAN_POINT ( 'NONE',  ( -4.566987299999997418, -46.89170807884566727, -98.39999999890753202 ) ) ;
#5504=COLOUR_RGB ( '', 0.09019608, 0.27058824, 0.51372549) ;
#5505=CARTESIAN_POINT ( 'NONE',  ( 2.071067811865474173, -39.99999999999997158, -99.24300000002186550 ) ) ;
#5510=PRODUCT_CONTEXT ( 'NONE', #8587, 'mechanical' ) ;
#5517=EDGE_CURVE ( 'NONE', #71, #7654, #4641, .T. ) ;
#5518=DIRECTION ( 'NONE',  ( -0.000000000000000000, -0.000000000000000000, -1.000000000000000000 ) ) ;
#5521=CARTESIAN_POINT ( 'NONE',  ( 2.071067811865477282, -49.99999999999997158, -99.44999999781505551 ) ) ;
#5525=VERTEX_POINT ( 'NONE', #6664 ) ;
#5531=CARTESIAN_POINT ( 'NONE',  ( -4.566987299999998307, -43.10829192115428299, -97.69999999890751496 ) ) ;
#5535=CARTESIAN_POINT ( 'NONE',  ( -4.566987299999998307, -43.10829192115428299, -97.89999999890751781 ) ) ;
#5537=FACE_OUTER_BOUND ( 'NONE', #614, .T. ) ;
#5544=CARTESIAN_POINT ( 'NONE',  ( -4.566987299999998307, -44.99999999999997158, -100.2499999989075121 ) ) ;
#5546=CARTESIAN_POINT ( 'NONE',  ( 9.184850993605145972E-16, -49.99999999999997158, -99.49999999781503845 ) ) ;
#5548=CARTESIAN_POINT ( 'NONE',  ( 4.566987299999998307, -44.99999999999997158, -97.24999999890752633 ) ) ;
#5550=CARTESIAN_POINT ( 'NONE',  ( 9.184850993605145972E-16, -49.99999999999997158, -95.60000000000000853 ) ) ;
#5552=CARTESIAN_POINT ( 'NONE',  ( 1.891708078845685481, -49.56698729999997255, -96.59999999890754907 ) ) ;
#5556=CARTESIAN_POINT ( 'NONE',  ( 5.000000000000000000, -47.07106781186545419, -100.1499999978150441 ) ) ;
#5563=ORIENTED_EDGE ( 'NONE', *, *, #2044, .F. ) ;
#5565=ORIENTED_EDGE ( 'NONE', *, *, #1671, .F. ) ;
#5572=CARTESIAN_POINT ( 'NONE',  ( 8.389419568037416259E-16, -49.56698729999997255, -95.84999999890753486 ) ) ;
#5573=CARTESIAN_POINT ( 'NONE',  ( -3.535533905932736864, -41.46446609406723383, -99.90000000000000568 ) ) ;
#5575=CARTESIAN_POINT ( 'NONE',  ( -3.229347689422839451, -48.22934768942280925, -96.14999999890753202 ) ) ;
#5583=VERTEX_POINT ( 'NONE', #3329 ) ;
#5586=CARTESIAN_POINT ( 'NONE',  ( -1.891708078845683039, -40.43301269999998482, -99.59999999890753486 ) ) ;
#5587=CARTESIAN_POINT ( 'NONE',  ( 2.071067811865474173, -39.99999999999997158, -99.94999999781505551 ) ) ;
#5589=CARTESIAN_POINT ( 'NONE',  ( 4.999999999999998224, -44.99999999999997158, -99.29999999781504982 ) ) ;
#5591=CARTESIAN_POINT ( 'NONE',  ( -1.891708078845683483, -49.56698729999997255, -99.09999999890753486 ) ) ;
#5592=VERTEX_POINT ( 'NONE', #4734 ) ;
#5595=ADVANCED_FACE ( 'NONE', ( #10 ), #2000, .T. ) ;
#5597=CARTESIAN_POINT ( 'NONE',  ( 9.184850993605145972E-16, -49.99999999999997158, -98.79300000002184845 ) ) ;
#5598=CARTESIAN_POINT ( 'NONE',  ( -2.796473189345805913E-16, -40.43301269999997061, -95.44999999890752918 ) ) ;
#5607=AXIS2_PLACEMENT_3D ( 'NONE', #6865, #4931, #5448 ) ;
#5609=CARTESIAN_POINT ( 'NONE',  ( 2.518094901854496914, -40.63106805822869205, -100.0000000000000142 ) ) ;
#5618=CARTESIAN_POINT ( 'NONE',  ( 4.566987300000000083, -46.89170807884564596, -97.29999999890752349 ) ) ;
#5621=CARTESIAN_POINT ( 'NONE',  ( -3.229347689422840784, -41.77065231057713390, -98.74999999890751212 ) ) ;
#5625=CARTESIAN_POINT ( 'NONE',  ( 0.000000000000000000, -44.99999999999997158, -95.00000000000000000 ) ) ;
#5626=ORIENTED_EDGE ( 'NONE', *, *, #1766, .T. ) ;
#5633=LINE ( 'NONE', #8381, #1337 ) ;
#5634=CARTESIAN_POINT ( 'NONE',  ( -2.071067811865475061, -39.99999999999997158, -100.6499999978150441 ) ) ;
#5636=CARTESIAN_POINT ( 'NONE',  ( -1.891708078845683039, -40.43301269999998482, -96.99999999890752633 ) ) ;
#5639=AXIS2_PLACEMENT_3D ( 'NONE', #38, #2742, #5410 ) ;
#5640=CARTESIAN_POINT ( 'NONE',  ( 2.071067811865477282, -49.99999999999996447, -99.54300000002184845 ) ) ;
#5643=CARTESIAN_POINT ( 'NONE',  ( 9.184850993605145972E-16, -49.99999999999997158, -96.29999999781504982 ) ) ;
#5646=CARTESIAN_POINT ( 'NONE',  ( 3.535533905932737309, -48.53553390593270933, -100.1999999978150555 ) ) ;
#5662=CARTESIAN_POINT ( 'NONE',  ( 4.566987299999998307, -44.99999999999997158, -98.04999999890752349 ) ) ;
#5663=CARTESIAN_POINT ( 'NONE',  ( -2.796473189345805913E-16, -40.43301269999997061, -100.4499999989075292 ) ) ;
#5666=CARTESIAN_POINT ( 'NONE',  ( -1.891708078845683483, -49.56698729999997255, -98.49999999890752633 ) ) ;
#5668=CARTESIAN_POINT ( 'NONE',  ( -4.999999999999998224, -44.99999999999997158, -95.34999999890753486 ) ) ;
#5669=CARTESIAN_POINT ( 'NONE',  ( 3.229347689422841228, -48.22934768942280925, -96.74999999890751212 ) ) ;
#5677=CARTESIAN_POINT ( 'NONE',  ( 4.999999999999998224, -44.99999999999997158, -96.20000000000000284 ) ) ;
#5678=CARTESIAN_POINT ( 'NONE',  ( -2.071067811865475061, -39.99999999999997158, -98.24999999781506688 ) ) ;
#5679=DIRECTION ( 'NONE',  ( -0.000000000000000000, -0.000000000000000000, -1.000000000000000000 ) ) ;
#5680=CARTESIAN_POINT ( 'NONE',  ( -2.071067811865475505, -49.99999999999996447, -97.25000000000000000 ) ) ;
#5687=CARTESIAN_POINT ( 'NONE',  ( -4.566987299999997418, -46.89170807884566727, -95.99999999890752633 ) ) ;
#5688=CARTESIAN_POINT ( 'NONE',  ( -4.999999999999997335, -47.07106781186546129, -97.24999999781506688 ) ) ;
#5690=DIRECTION ( 'NONE',  ( -1.000000000000000000, 0.000000000000000000, 0.000000000000000000 ) ) ;
#5705=CARTESIAN_POINT ( 'NONE',  ( -2.796473189345805913E-16, -40.43301269999997061, -98.64999999890753202 ) ) ;
#5710=CARTESIAN_POINT ( 'NONE',  ( 4.566987299999998307, -43.10829192115428299, -99.79999999890752349 ) ) ;
#5713=CARTESIAN_POINT ( 'NONE',  ( 3.229347689422839895, -41.77065231057713390, -96.54999999890752349 ) ) ;
#5721=CARTESIAN_POINT ( 'NONE',  ( 4.566987299999998307, -44.99999999999997158, -99.84999999890752065 ) ) ;
#5722=CARTESIAN_POINT ( 'NONE',  ( 4.999999999999998224, -44.99999999999997158, -95.40000000000000568 ) ) ;
#5725=CARTESIAN_POINT ( 'NONE',  ( 3.535533905932737309, -48.53553390593270933, -96.29999999999999716 ) ) ;
#5732=CARTESIAN_POINT ( 'NONE',  ( 5.000000000000000000, -47.07106781186545419, -98.65000000000000568 ) ) ;
#5733=CARTESIAN_POINT ( 'NONE',  ( -4.999999999999998224, -42.92893218813448897, -97.34999999781506119 ) ) ;
#5741=DIRECTION ( 'NONE',  ( 0.000000000000000000, 0.000000000000000000, -1.000000000000000000 ) ) ;
#5746=VERTEX_POINT ( 'NONE', #4636 ) ;
#5750=CARTESIAN_POINT ( 'NONE',  ( -4.566987299999998307, -44.99999999999997158, -98.44999999890752918 ) ) ;
#5753=FACE_OUTER_BOUND ( 'NONE', #1867, .T. ) ;
#5755=CARTESIAN_POINT ( 'NONE',  ( 3.229347689422841228, -48.22934768942280925, -98.34999999890752065 ) ) ;
#5764=CYLINDRICAL_SURFACE ( 'NONE', #6303, 4.999999999999998224 ) ;
#5768=CARTESIAN_POINT ( 'NONE',  ( 4.999999999999998224, -42.92893218813448897, -95.34999999999999432 ) ) ;
#5774=CARTESIAN_POINT ( 'NONE',  ( 2.071067811865477282, -49.99999999999996447, -96.35000000000000853 ) ) ;
#5776=CARTESIAN_POINT ( 'NONE',  ( -3.061616997868382155E-16, -39.99999999999997158, -95.89999999781505835 ) ) ;
#5781=CARTESIAN_POINT ( 'NONE',  ( -3.535533905932736864, -41.46446609406723383, -99.79999999781504982 ) ) ;
#5798=CARTESIAN_POINT ( 'NONE',  ( 4.566987299999998307, -44.99999999999997158, -97.44999999890751496 ) ) ;
#5806=AXIS2_PLACEMENT_3D ( 'NONE', #175, #1534, #6957 ) ;
#5808=( BOUNDED_SURFACE ( )  B_SPLINE_SURFACE ( 1, 2, ( 
 ( #6963, #3666, #7054, #2308, #5598, #6346, #8300, #928, #1497, #133, #3622, #7670, #1013, #309, #8216, #5687, #8389, #3709, #2350, #180, #2833, #4192, #6874, #2261, #836, #3539, #6217, #5552, #8258, #2219, #4902, #7581, #1542, #4237, #2788, #5636, #1492, #4807, #8336, #4983, #5548, #176, #3491, #2301, #5453, #875, #7665, #2169, #2213, #3534, #1626, #2828, #4147, #6869, #2124, #6299, #129, #6825, #789, #7532, #2919, #4319, #259, #5501, #2257, #3577, #7003, #4230, #6173, #8253, #6261, #6958, #965, #6212, #832, #1582, #2875, #5591, #2962, #8210, #4855, #4897, #217, #8296, #4935, #7575, #4189, #1535, #6125, #6913, #8164, #7617, #4275, #922, #7489, #81, #3618, #1454, #304, #2390, #2468 ),
 ( #4406, #7841, #7094, #420, #3830, #3703, #1674, #5768, #1096, #3135, #5151, #6428, #1006, #384, #3661, #8467, #3006, #1808, #8506, #2343, #3090, #1052, #7047, #7218, #7800, #2429, #5725, #2513, #5108, #1768, #4449, #3744, #4364, #8384, #5189, #3790, #4489, #343, #7133, #5813, #6384, #7885, #6467, #1135, #5065, #5680, #3051, #7174, #6509, #1850, #462, #8426, #3177, #5854, #8546, #4533, #6340, #5024, #7715, #7755, #1720, #6683, #1259, #1933, #8714, #5900, #2643, #7349, #7259, #2552, #4619, #4660, #3348, #4047, #4710, #5314, #28, #1181, #8015, #1304, #8633, #5939, #1972, #3258, #4003, #6636, #594, #7970, #6552, #687, #5269, #8585, #3393, #2729, #3307, #3958, #1220, #6069, #503, #641, #5399 ) ),
 .UNSPECIFIED., .F., .F., .T. ) 
 B_SPLINE_SURFACE_WITH_KNOTS ( ( 2, 2 ),
 ( 3, 2, 2, 2, 2, 2, 2, 2, 2, 2, 2, 2, 2, 2, 2, 2, 2, 2, 2, 2, 2, 2, 2, 2, 2, 2, 2, 2, 2, 2, 2, 2, 2, 2, 2, 2, 2, 2, 2, 2, 2, 2, 2, 2, 2, 2, 2, 2, 2, 2, 3 ),
 ( 0.000000000000000000, 1.000000000000000000 ),
 ( 0.000000000000000000, 0.01785714285714285615, 0.03571428571428571230, 0.05357142857142856845, 0.07142857142857142461, 0.08928571428571428770, 0.1071428571428571369, 0.1250000000000000000, 0.1428571428571428492, 0.1607142857142857262, 0.1785714285714285754, 0.1964285714285714246, 0.2142857142857142738, 0.2321428571428571508, 0.2500000000000000000, 0.2678571428571428492, 0.2857142857142856984, 0.3035714285714285476, 0.3214285714285714524, 0.3392857142857143016, 0.3571428571428571508, 0.3750000000000000000, 0.3928571428571428492, 0.4107142857142856984, 0.4285714285714285476, 0.4464285714285714524, 0.4642857142857143016, 0.4821428571428571508, 0.5000000000000000000, 0.5178571428571429047, 0.5357142857142856984, 0.5535714285714286031, 0.5714285714285713969, 0.5892857142857143016, 0.6071428571428570953, 0.6250000000000000000, 0.6428571428571429047, 0.6607142857142856984, 0.6785714285714286031, 0.6964285714285713969, 0.7142857142857143016, 0.7321428571428570953, 0.7500000000000000000, 0.7678571428571429047, 0.7857142857142856984, 0.8035714285714286031, 0.8214285714285713969, 0.8392857142857143016, 0.8571428571428570953, 0.8750000000000000000, 0.8928571428571429047 ),
 .UNSPECIFIED. ) 
 GEOMETRIC_REPRESENTATION_ITEM ( )  RATIONAL_B_SPLINE_SURFACE ( (
 ( 1.000000000000000000, 0.9238795325112867385, 1.000000000000000000, 0.9238795325112867385, 1.000000000000000000, 0.9238795325112867385, 1.000000000000000000, 0.9238795325112867385, 1.000000000000000000, 0.9238795325112867385, 1.000000000000000000, 0.9238795325112867385, 1.000000000000000000, 0.9238795325112867385, 1.000000000000000000, 0.9238795325112867385, 1.000000000000000000, 0.9238795325112867385, 1.000000000000000000, 0.9238795325112867385, 1.000000000000000000, 0.9238795325112867385, 1.000000000000000000, 0.9238795325112867385, 1.000000000000000000, 0.9238795325112867385, 1.000000000000000000, 0.9238795325112867385, 1.000000000000000000, 0.9238795325112867385, 1.000000000000000000, 0.9238795325112867385, 1.000000000000000000, 0.9238795325112867385, 1.000000000000000000, 0.9238795325112867385, 1.000000000000000000, 0.9238795325112867385, 1.000000000000000000, 0.9238795325112867385, 1.000000000000000000, 0.9238795325112867385, 1.000000000000000000, 0.9238795325112867385, 1.000000000000000000, 0.9238795325112867385, 1.000000000000000000, 0.9238795325112867385, 1.000000000000000000, 0.9238795325112867385, 1.000000000000000000, 0.9238795325112867385, 1.000000000000000000, 0.9238795325112867385, 1.000000000000000000, 0.9238795325112867385, 1.000000000000000000, 0.9238795325112867385, 1.000000000000000000, 0.9238795325112867385, 1.000000000000000000, 0.9238795325112867385, 1.000000000000000000, 0.9238795325112867385, 1.000000000000000000, 0.9238795325112867385, 1.000000000000000000, 0.9238795325112867385, 1.000000000000000000, 0.9238795325112867385, 1.000000000000000000, 0.9238795325112867385, 1.000000000000000000, 0.9238795325112867385, 1.000000000000000000, 0.9238795325112867385, 1.000000000000000000, 0.9238795325112867385, 1.000000000000000000, 0.9238795325112867385, 1.000000000000000000, 0.9238795325112867385, 1.000000000000000000, 0.9238795325112867385, 1.000000000000000000, 0.9238795325112867385, 1.000000000000000000, 0.9238795325112867385, 1.000000000000000000, 0.9238795325112867385, 1.000000000000000000, 0.9238795325112867385, 1.000000000000000000, 0.9238795325112867385, 1.000000000000000000, 0.9238795325112867385, 1.000000000000000000, 0.9238795325112867385, 1.000000000000000000, 0.9238795325112867385, 1.000000000000000000),
 ( 1.000000000000000000, 0.9238795325112867385, 1.000000000000000000, 0.9238795325112867385, 1.000000000000000000, 0.9238795325112867385, 1.000000000000000000, 0.9238795325112867385, 1.000000000000000000, 0.9238795325112867385, 1.000000000000000000, 0.9238795325112867385, 1.000000000000000000, 0.9238795325112867385, 1.000000000000000000, 0.9238795325112867385, 1.000000000000000000, 0.9238795325112867385, 1.000000000000000000, 0.9238795325112867385, 1.000000000000000000, 0.9238795325112867385, 1.000000000000000000, 0.9238795325112867385, 1.000000000000000000, 0.9238795325112867385, 1.000000000000000000, 0.9238795325112867385, 1.000000000000000000, 0.9238795325112867385, 1.000000000000000000, 0.9238795325112867385, 1.000000000000000000, 0.9238795325112867385, 1.000000000000000000, 0.9238795325112867385, 1.000000000000000000, 0.9238795325112867385, 1.000000000000000000, 0.9238795325112867385, 1.000000000000000000, 0.9238795325112867385, 1.000000000000000000, 0.9238795325112867385, 1.000000000000000000, 0.9238795325112867385, 1.000000000000000000, 0.9238795325112867385, 1.000000000000000000, 0.9238795325112867385, 1.000000000000000000, 0.9238795325112867385, 1.000000000000000000, 0.9238795325112867385, 1.000000000000000000, 0.9238795325112867385, 1.000000000000000000, 0.9238795325112867385, 1.000000000000000000, 0.9238795325112867385, 1.000000000000000000, 0.9238795325112867385, 1.000000000000000000, 0.9238795325112867385, 1.000000000000000000, 0.9238795325112867385, 1.000000000000000000, 0.9238795325112867385, 1.000000000000000000, 0.9238795325112867385, 1.000000000000000000, 0.9238795325112867385, 1.000000000000000000, 0.9238795325112867385, 1.000000000000000000, 0.9238795325112867385, 1.000000000000000000, 0.9238795325112867385, 1.000000000000000000, 0.9238795325112867385, 1.000000000000000000, 0.9238795325112867385, 1.000000000000000000, 0.9238795325112867385, 1.000000000000000000, 0.9238795325112867385, 1.000000000000000000, 0.9238795325112867385, 1.000000000000000000, 0.9238795325112867385, 1.000000000000000000, 0.9238795325112867385, 1.000000000000000000, 0.9238795325112867385, 1.000000000000000000, 0.9238795325112867385, 1.000000000000000000, 0.9238795325112867385, 1.000000000000000000, 0.9238795325112867385, 1.000000000000000000) ) ) 
 REPRESENTATION_ITEM ( '' )  SURFACE ( )  );
#5809=CYLINDRICAL_SURFACE ( 'NONE', #7006, 4.999999999999998224 ) ;
#5811=CARTESIAN_POINT ( 'NONE',  ( 9.184850993605145972E-16, -49.99999999999997158, -97.19999999999998863 ) ) ;
#5813=CARTESIAN_POINT ( 'NONE',  ( 4.999999999999998224, -42.92893218813448897, -96.95000000000000284 ) ) ;
#5821=CARTESIAN_POINT ( 'NONE',  ( 4.999999999999998224, -44.99999999999997158, -97.79999999999999716 ) ) ;
#5823=CARTESIAN_POINT ( 'NONE',  ( 3.535533969928884801, -41.46446615806338087, -100.0000000000000142 ) ) ;
#5827=CARTESIAN_POINT ( 'NONE',  ( -4.999999999999998224, -44.99999999999997158, -97.29999999781504982 ) ) ;
#5828=DIRECTION ( 'NONE',  ( -1.000000000000000000, 0.000000000000000000, 0.000000000000000000 ) ) ;
#5835=CARTESIAN_POINT ( 'NONE',  ( 3.229347689422839895, -41.77065231057713390, -98.74999999890752633 ) ) ;
#5840=DIRECTION ( 'NONE',  ( -0.000000000000000000, -0.000000000000000000, 1.000000000000000000 ) ) ;
#5841=CARTESIAN_POINT ( 'NONE',  ( -3.229347689422839451, -48.22934768942280925, -96.14999999890753202 ) ) ;
#5842=DIRECTION ( 'NONE',  ( -1.000000000000000000, 0.000000000000000000, 0.000000000000000000 ) ) ;
#5850=CARTESIAN_POINT ( 'NONE',  ( 0.000000000000000000, -44.99999999999997158, -105.0000000000000142 ) ) ;
#5853=CARTESIAN_POINT ( 'NONE',  ( -7.499999999999999112, -44.99999999999997158, -100.0000000000000000 ) ) ;
#5854=CARTESIAN_POINT ( 'NONE',  ( 2.071067811865474173, -39.99999999999997158, -97.64999999999999147 ) ) ;
#5862=CARTESIAN_POINT ( 'NONE',  ( 2.071067811865477282, -49.99999999999996447, -97.95000000000000284 ) ) ;
#5863=CARTESIAN_POINT ( 'NONE',  ( -1.135448125450190027, -40.09623321959037412, -100.0007921917414109 ) ) ;
#5864=EDGE_CURVE ( 'NONE', #5143, #7654, #4008, .T. ) ;
#5874=PRODUCT_DEFINITION ( 'UNKNOWN', '', #7062, #2218 ) ;
#5880=CARTESIAN_POINT ( 'NONE',  ( 8.389419568037416259E-16, -49.56698729999997255, -99.84999999890753486 ) ) ;
#5885=CARTESIAN_POINT ( 'NONE',  ( -4.999999999999998224, -42.92893218813449607, -98.94999999781505551 ) ) ;
#5888=CARTESIAN_POINT ( 'NONE',  ( -4.566987299999998307, -43.10829192115428299, -98.69999999890752918 ) ) ;
#5898=CARTESIAN_POINT ( 'NONE',  ( -3.535533905932735532, -48.53553390593270933, -97.29999999999999716 ) ) ;
#5899=CARTESIAN_POINT ( 'NONE',  ( -2.071067811865475505, -49.99999999999997158, -96.45000000000000284 ) ) ;
#5900=CARTESIAN_POINT ( 'NONE',  ( -4.999999999999998224, -42.92893218813448897, -98.25000000000000000 ) ) ;
#5905=DIRECTION ( 'NONE',  ( -0.000000000000000000, -0.000000000000000000, -1.000000000000000000 ) ) ;
#5906=CARTESIAN_POINT ( 'NONE',  ( 3.535533905932736420, -41.46446609406723383, -96.10000000000000853 ) ) ;
#5908=CARTESIAN_POINT ( 'NONE',  ( -2.944777139751900918, -49.07987410177226906, -100.0011278004036797 ) ) ;
#5910=( BOUNDED_CURVE ( )  B_SPLINE_CURVE ( 2, ( #4726, #2222, #7497, #1459, #6040, #3410, #6876, #7410, #4771 ),
 .UNSPECIFIED., .F., .T. ) 
 B_SPLINE_CURVE_WITH_KNOTS ( ( 3, 2, 2, 2, 3 ),
 ( 0.000000000000000000, 0.01785714285714282840, 0.03571428571428565679, 0.05357142857142848519, 0.07142857142857131358 ),
 .UNSPECIFIED. ) 
 CURVE ( )  GEOMETRIC_REPRESENTATION_ITEM ( )  RATIONAL_B_SPLINE_CURVE ( ( 1.000000000000000000, 0.9238795325112867385, 1.000000000000000000, 0.9238795325112867385, 1.000000000000000000, 0.9238795325112867385, 1.000000000000000000, 0.9238795325112871826, 0.9999999999999995559 ) ) 
 REPRESENTATION_ITEM ( '' )  );
#5911=CARTESIAN_POINT ( 'NONE',  ( 2.071067811865474173, -39.99999999999997158, -99.94999999781505551 ) ) ;
#5925=CARTESIAN_POINT ( 'NONE',  ( -3.061616997868382155E-16, -39.99999999999997158, -99.09999999781504698 ) ) ;
#5927=CARTESIAN_POINT ( 'NONE',  ( -4.566987299999998307, -44.99999999999997158, -98.64999999890751781 ) ) ;
#5936=CARTESIAN_POINT ( 'NONE',  ( 2.071067811865474173, -39.99999999999997158, -99.25000000000000000 ) ) ;
#5937=CARTESIAN_POINT ( 'NONE',  ( 9.184850993605145972E-16, -49.99999999999997158, -99.49999999781503845 ) ) ;
#5939=CARTESIAN_POINT ( 'NONE',  ( -4.999999999999998224, -42.92893218813448897, -99.05000000000001137 ) ) ;
#5946=CARTESIAN_POINT ( 'NONE',  ( 4.999999999999998224, -42.92893218813448897, -97.64999999781504414 ) ) ;
#5948=CARTESIAN_POINT ( 'NONE',  ( 4.566987299999998307, -44.99999999999997158, -99.64999999890753202 ) ) ;
#5950=CARTESIAN_POINT ( 'NONE',  ( -3.760469397705862526, -48.30756035107769719, -99.99941978915393292 ) ) ;
#5952=VECTOR ( 'NONE', #5219, 1000.000000000000000 ) ;
#5953=CARTESIAN_POINT ( 'NONE',  ( -4.999999999999998224, -42.92893218813448897, -97.44300000002183992 ) ) ;
#5966=CARTESIAN_POINT ( 'NONE',  ( 3.535533905932736420, -41.46446609406723383, -99.19999999781505551 ) ) ;
#5968=CARTESIAN_POINT ( 'NONE',  ( -4.566987299999998307, -44.99999999999997158, -95.24999999890752633 ) ) ;
#5975=EDGE_LOOP ( 'NONE', ( #2921, #6991, #3833, #816, #8184, #5626, #3947, #8034, #6959, #29, #8580, #6116, #421, #6730, #1825, #5565 ) ) ;
#5979=CARTESIAN_POINT ( 'NONE',  ( 4.999999999999998224, -44.99999999999997158, -98.49999999781503845 ) ) ;
#5987=CARTESIAN_POINT ( 'NONE',  ( 1.891708078845682595, -40.43301269999998482, -98.89999999890751781 ) ) ;
#5988=CARTESIAN_POINT ( 'NONE',  ( -4.999999999999998224, -42.92893218813448897, -95.74999999781503845 ) ) ;
#5990=CARTESIAN_POINT ( 'NONE',  ( -3.229347689422839451, -48.22934768942280925, -99.94999999890752918 ) ) ;
#5993=CARTESIAN_POINT ( 'NONE',  ( -4.999999999999998224, -44.99999999999997158, -94.99300000002185129 ) ) ;
#5997=CARTESIAN_POINT ( 'NONE',  ( -4.999999999999998224, -44.99999999999997158, -95.79999999999999716 ) ) ;
#6004=CARTESIAN_POINT ( 'NONE',  ( 2.071067811865474173, -39.99999999999997158, -96.85000000000002274 ) ) ;
#6010=CARTESIAN_POINT ( 'NONE',  ( 1.891708078845685481, -49.56698729999997255, -99.99999999890751212 ) ) ;
#6011=AXIS2_PLACEMENT_3D ( 'NONE', #5850, #3086, #6336 ) ;
#6023=CARTESIAN_POINT ( 'NONE',  ( 5.000000000000000000, -47.07106781186545419, -100.1499999978150441 ) ) ;
#6026=EDGE_LOOP ( 'NONE', ( #707, #3040, #2939 ) ) ;
#6027=EDGE_CURVE ( 'NONE', #2692, #7413, #7996, .T. ) ;
#6031=CARTESIAN_POINT ( 'NONE',  ( -3.229347689422839451, -48.22934768942280925, -99.34999999890752065 ) ) ;
#6032=CARTESIAN_POINT ( 'NONE',  ( -4.999999999999998224, -44.99999999999997158, -99.79999999999999716 ) ) ;
#6034=CARTESIAN_POINT ( 'NONE',  ( -1.891708078845683483, -49.56698729999997255, -99.89999999890753202 ) ) ;
#6036=CARTESIAN_POINT ( 'NONE',  ( 5.000000000000000000, -47.07106781186545419, -97.04300000002184845 ) ) ;
#6039=CARTESIAN_POINT ( 'NONE',  ( -3.061616997868382155E-16, -39.99999999999997158, -97.60000000000000853 ) ) ;
#6040=CARTESIAN_POINT ( 'NONE',  ( -3.061616997868382155E-16, -39.99999999999997158, -95.89999999781505835 ) ) ;
#6052=CARTESIAN_POINT ( 'NONE',  ( -3.229347689422840784, -41.77065231057713390, -98.74999999890751212 ) ) ;
#6061=COLOUR_RGB ( '', 0.09019608, 0.27058824, 0.51372549) ;
#6063=ORIENTED_EDGE ( 'NONE', *, *, #2221, .T. ) ;
#6067=CARTESIAN_POINT ( 'NONE',  ( -3.535533905932736864, -41.46446609406723383, -98.99999999781503845 ) ) ;
#6069=CARTESIAN_POINT ( 'NONE',  ( -4.999999999999998224, -42.92893218813448897, -99.85000000000002274 ) ) ;
#6076=CARTESIAN_POINT ( 'NONE',  ( -1.891708078845683039, -40.43301269999998482, -98.79999999890750928 ) ) ;
#6077=CARTESIAN_POINT ( 'NONE',  ( 3.535533905932737309, -48.53553390593270933, -96.99999999781503845 ) ) ;
#6079=CARTESIAN_POINT ( 'NONE',  ( 4.566987299999998307, -44.99999999999997158, -97.24999999890752633 ) ) ;
#6080=FACE_OUTER_BOUND ( 'NONE', #8579, .T. ) ;
#6084=CARTESIAN_POINT ( 'NONE',  ( 5.000000000000000000, -47.07106781186545419, -97.84300000002187403 ) ) ;
#6097=CARTESIAN_POINT ( 'NONE',  ( -3.535533905932736864, -41.46446609406723383, -98.99999999781503845 ) ) ;
#6099=VERTEX_POINT ( 'NONE', #5033 ) ;
#6104=AXIS2_PLACEMENT_3D ( 'NONE', #3479, #1524, #6161 ) ;
#6111=CARTESIAN_POINT ( 'NONE',  ( 4.566987299999998307, -44.99999999999997158, -95.84999999890752065 ) ) ;
#6116=ORIENTED_EDGE ( 'NONE', *, *, #916, .T. ) ;
#6121=CARTESIAN_POINT ( 'NONE',  ( -4.566987299999998307, -43.10829192115428299, -97.09999999890752065 ) ) ;
#6122=ADVANCED_FACE ( 'NONE', ( #5120 ), #3145, .T. ) ;
#6123=CARTESIAN_POINT ( 'NONE',  ( 9.184850993605145972E-16, -49.99999999999997158, -97.89999999781504414 ) ) ;
#6125=CARTESIAN_POINT ( 'NONE',  ( 4.566987299999998307, -44.99999999999997158, -99.64999999890753202 ) ) ;
#6128=CARTESIAN_POINT ( 'NONE',  ( -2.071067811865475505, -49.99999999999996447, -97.24300000002185129 ) ) ;
#6132=ADVANCED_FACE ( 'NONE', ( #7812 ), #6477, .T. ) ;
#6140=( BOUNDED_CURVE ( )  B_SPLINE_CURVE ( 2, ( #3533, #6211, #7574, #8163, #921, #4934, #1453, #7616, #258 ),
 .UNSPECIFIED., .F., .T. ) 
 B_SPLINE_CURVE_WITH_KNOTS ( ( 3, 2, 2, 2, 3 ),
 ( 0.3571428571428572063, 0.3750000000000000000, 0.3928571428571427937, 0.4107142857142856429, 0.4285714285714284366 ),
 .UNSPECIFIED. ) 
 CURVE ( )  GEOMETRIC_REPRESENTATION_ITEM ( )  RATIONAL_B_SPLINE_CURVE ( ( 0.9999999999999997780, 0.9238795325112869605, 1.000000000000000000, 0.9238795325112867385, 1.000000000000000000, 0.9238795325112867385, 1.000000000000000000, 0.9238795325112871826, 0.9999999999999995559 ) ) 
 REPRESENTATION_ITEM ( '' )  );
#6147=VECTOR ( 'NONE', #4640, 1000.000000000000000 ) ;
#6150=VERTEX_POINT ( 'NONE', #1683 ) ;
#6157=CARTESIAN_POINT ( 'NONE',  ( -2.796473189345805913E-16, -40.43301269999997061, -95.44999999890752918 ) ) ;
#6160=CARTESIAN_POINT ( 'NONE',  ( -2.796473189345805913E-16, -40.43301269999997061, -96.44999999890751496 ) ) ;
#6161=DIRECTION ( 'NONE',  ( -1.000000000000000000, 0.000000000000000000, 0.000000000000000000 ) ) ;
#6163=ORIENTED_EDGE ( 'NONE', *, *, #1743, .F. ) ;
#6169=CYLINDRICAL_SURFACE ( 'NONE', #5607, 4.999999999999998224 ) ;
#6170=CARTESIAN_POINT ( 'NONE',  ( -4.566987299999997418, -46.89170807884566017, -98.59999999890753486 ) ) ;
#6171=CARTESIAN_POINT ( 'NONE',  ( -3.535533905932735532, -48.53553390593270933, -99.59999999781504698 ) ) ;
#6173=CARTESIAN_POINT ( 'NONE',  ( -2.796473189345805913E-16, -40.43301269999997061, -98.64999999890753202 ) ) ;
#6175=CARTESIAN_POINT ( 'NONE',  ( 3.535533905932737309, -48.53553390593270933, -95.50000000000000000 ) ) ;
#6196=ORIENTED_EDGE ( 'NONE', *, *, #7701, .F. ) ;
#6197=CARTESIAN_POINT ( 'NONE',  ( 1.891708078845685481, -49.56698729999997255, -96.59999999890754907 ) ) ;
#6199=CARTESIAN_POINT ( 'NONE',  ( 4.566987299999998307, -44.99999999999997158, -98.24999999890751212 ) ) ;
#6207=CARTESIAN_POINT ( 'NONE',  ( 9.184850993605145972E-16, -49.99999999999997158, -98.69999999781505551 ) ) ;
#6208=CARTESIAN_POINT ( 'NONE',  ( -4.566987299999998307, -43.10829192115428299, -99.49999999890752633 ) ) ;
#6209=CARTESIAN_POINT ( 'NONE',  ( -4.999999999999997335, -47.07106781186546129, -98.84999999781503277 ) ) ;
#6211=CARTESIAN_POINT ( 'NONE',  ( 4.999999999999994671, -47.07106781186546129, -97.74999999781505267 ) ) ;
#6212=CARTESIAN_POINT ( 'NONE',  ( 4.566987300000000083, -46.89170807884565306, -98.89999999890753202 ) ) ;
#6215=CARTESIAN_POINT ( 'NONE',  ( -4.999999999999998224, -44.99999999999997158, -98.99300000002185129 ) ) ;
#6217=CARTESIAN_POINT ( 'NONE',  ( 3.229347689422841228, -48.22934768942280925, -96.54999999890752349 ) ) ;
#6219=CARTESIAN_POINT ( 'NONE',  ( 4.566987299999998307, -43.10829192115428299, -96.59999999890753486 ) ) ;
#6242=CARTESIAN_POINT ( 'NONE',  ( 3.229347689422839895, -41.77065231057713390, -95.54999999890752349 ) ) ;
#6247=CARTESIAN_POINT ( 'NONE',  ( 4.566987299999998307, -43.10829192115428299, -98.19999999890751496 ) ) ;
#6249=DIRECTION ( 'NONE',  ( -0.000000000000000000, -0.000000000000000000, -1.000000000000000000 ) ) ;
#6251=VERTEX_POINT ( 'NONE', #8475 ) ;
#6259=CARTESIAN_POINT ( 'NONE',  ( 2.071067811865474173, -39.99999999999997158, -98.34999999781506119 ) ) ;
#6261=CARTESIAN_POINT ( 'NONE',  ( 3.229347689422839895, -41.77065231057713390, -98.74999999890752633 ) ) ;
#6264=CARTESIAN_POINT ( 'NONE',  ( -2.071067811865475061, -39.99999999999997158, -99.14300000002185698 ) ) ;
#6274=ORIENTED_EDGE ( 'NONE', *, *, #8610, .F. ) ;
#6282=CARTESIAN_POINT ( 'NONE',  ( 1.891708078845682595, -40.43301269999998482, -95.49999999890754054 ) ) ;
#6283=DIRECTION ( 'NONE',  ( -0.000000000000000000, -0.000000000000000000, -1.000000000000000000 ) ) ;
#6284=CARTESIAN_POINT ( 'NONE',  ( 3.229347689422839895, -41.77065231057713390, -98.14999999890751781 ) ) ;
#6285=CARTESIAN_POINT ( 'NONE',  ( 5.000000000000000888, -42.92893218813449607, -95.34999999999999432 ) ) ;
#6287=( LENGTH_UNIT ( ) NAMED_UNIT ( * ) SI_UNIT ( .MILLI., .METRE. ) );
#6296=CARTESIAN_POINT ( 'NONE',  ( -4.999999999999997335, -47.07106781186546129, -98.04999999781504982 ) ) ;
#6299=CARTESIAN_POINT ( 'NONE',  ( 4.566987299999998307, -43.10829192115428299, -97.99999999890754054 ) ) ;
#6303=AXIS2_PLACEMENT_3D ( 'NONE', #8462, #2424, #299 ) ;
#6304=CARTESIAN_POINT ( 'NONE',  ( -4.999999999999998224, -42.92893218813448897, -95.04999999999999716 ) ) ;
#6306=CARTESIAN_POINT ( 'NONE',  ( 5.000000000000000000, -47.07106781186545419, -96.14999999781504414 ) ) ;
#6319=VERTEX_POINT ( 'NONE', #5589 ) ;
#6323=CARTESIAN_POINT ( 'NONE',  ( -3.229347689422840784, -41.77065231057713390, -97.74999999890752633 ) ) ;
#6324=CARTESIAN_POINT ( 'NONE',  ( -3.229347689422840784, -41.77065231057713390, -97.94999999890751496 ) ) ;
#6326=CARTESIAN_POINT ( 'NONE',  ( -1.891708078845683483, -49.56698729999997255, -96.09999999890750644 ) ) ;
#6328=ORIENTED_EDGE ( 'NONE', *, *, #2086, .T. ) ;
#6336=DIRECTION ( 'NONE',  ( 1.000000000000000000, 0.000000000000000000, 0.000000000000000000 ) ) ;
#6338=CARTESIAN_POINT ( 'NONE',  ( 2.071067811865477282, -49.99999999999996447, -98.64999999781504414 ) ) ;
#6340=CARTESIAN_POINT ( 'NONE',  ( 4.999999999999998224, -44.99999999999997158, -97.79999999999999716 ) ) ;
#6345=CARTESIAN_POINT ( 'NONE',  ( -4.999999999999998224, -44.99999999999997158, -98.19300000002183992 ) ) ;
#6346=CARTESIAN_POINT ( 'NONE',  ( 1.891708078845682595, -40.43301269999998482, -95.49999999890754054 ) ) ;
#6347=CARTESIAN_POINT ( 'NONE',  ( -3.061616997868382155E-16, -39.99999999999997158, -96.69999999781504130 ) ) ;
#6369=CARTESIAN_POINT ( 'NONE',  ( -4.566987299999997418, -46.89170807884566727, -99.39999999890751781 ) ) ;
#6371=CARTESIAN_POINT ( 'NONE',  ( 8.389419568037416259E-16, -49.56698729999997255, -96.84999999890752065 ) ) ;
#6372=DIRECTION ( 'NONE',  ( -0.000000000000000000, -0.000000000000000000, -1.000000000000000000 ) ) ;
#6380=DIRECTION ( 'NONE',  ( 0.000000000000000000, 0.000000000000000000, 1.000000000000000000 ) ) ;
#6384=CARTESIAN_POINT ( 'NONE',  ( 4.999999999999998224, -44.99999999999997158, -97.00000000000000000 ) ) ;
#6388=EDGE_CURVE ( 'NONE', #876, #6150, #6140, .T. ) ;
#6390=CARTESIAN_POINT ( 'NONE',  ( -2.071067811865475505, -49.99999999999996447, -98.04999999999999716 ) ) ;
#6391=CARTESIAN_POINT ( 'NONE',  ( 3.535533905932737309, -48.53553390593270933, -97.79999999781504982 ) ) ;
#6394=EDGE_CURVE ( 'NONE', #7878, #6586, #4677, .T. ) ;
#6402=DIRECTION ( 'NONE',  ( -0.000000000000000000, -0.000000000000000000, -1.000000000000000000 ) ) ;
#6405=ORIENTED_EDGE ( 'NONE', *, *, #8610, .T. ) ;
#6409=DIRECTION ( 'NONE',  ( -0.000000000000000000, -0.000000000000000000, -1.000000000000000000 ) ) ;
#6414=CARTESIAN_POINT ( 'NONE',  ( 3.229347689422839895, -41.77065231057713390, -98.14999999890751781 ) ) ;
#6415=CARTESIAN_POINT ( 'NONE',  ( -3.061616997868382155E-16, -39.99999999999997158, -100.6999999978150555 ) ) ;
#6419=EDGE_CURVE ( 'NONE', #4083, #6251, #6466, .T. ) ;
#6420=ORIENTED_EDGE ( 'NONE', *, *, #6419, .T. ) ;
#6422=( BOUNDED_SURFACE ( )  B_SPLINE_SURFACE ( 1, 2, ( 
 ( #5160, #3319, #5993, #747, #7407, #4105, #1989, #5413, #1364, #7317, #5327, #2612, #6740, #2082, #5458, #2792, #2035, #2746, #2658, #6605, #8123, #4063, #700, #7273, #4722, #4676, #7364, #6783, #3930, #1233, #4767, #1272, #3452, #8685, #1903, #88, #3972, #6695, #8027, #3363, #4589, #1318, #3406, #6036, #561, #8075, #6652, #6128, #1409, #3274, #7452, #5953, #7986, #607, #4630, #4017, #8646, #656, #5279, #6084, #1945, #1998, #2700, #5369, #42, #879, #6345, #2966, #970, #8299, #132, #2260, #2306, #2130, #4811, #7579, #4942, #4151, #5597, #3581, #7007, #4280, #6215, #1540, #6828, #6264, #7622, #5505, #794, #179, #2923, #1586, #4987, #5640, #221, #3665, #6962, #1632, #8257, #8341, #927, #4858, #2878, #2831, #3621 ),
 ( #7668, #308, #3537, #6304, #3496, #835, #4325, #3010, #264, #8167, #7495, #1457, #6175, #8214, #5550, #2171, #7535, #4235, #1495, #2217, #6916, #4901, #4191, #6873, #5906, #2434, #2474, #1227, #3834, #5774, #8594, #2559, #7931, #3880, #5236, #3750, #8471, #388, #8512, #6559, #5115, #7266, #5194, #1728, #2394, #3224, #5156, #3794, #7847, #4582, #1186, #1898, #6515, #7100, #468, #512, #347, #3055, #5821, #3182, #5070, #5862, #1813, #6390, #2518, #4454, #4494, #7761, #7182, #8554, #6435, #4413, #7139, #1141, #7890, #5732, #8430, #1857, #1057, #3094, #4538, #7223, #7807, #1773, #1101, #6473, #426, #3141, #4056, #694, #5321, #3924, #741, #648, #7445, #4669, #3357, #2785, #6032, #6643, #8640, #1266, #2606, #4099, #6776 ),
 ( #4804, #600, #2652, #5988, #79, #4625, #5274, #7309, #8021, #1981, #5450, #8162, #3966, #1403, #7357, #6735, #2122, #5226, #3266, #3400, #5363, #7487, #3446, #3314, #8116, #6599, #7978, #2694, #6077, #1940, #8066, #8679, #1311, #35, #2029, #4011, #4717, #6690, #7401, #1356, #2738, #5946, #554, #5407, #2074, #4761, #6123, #2299, #8294, #6296, #920, #3658, #8333, #5678, #3616, #6259, #7530, #2341, #4186, #174, #3532, #6338, #2167, #2255, #2960, #6209, #1452, #873, #1624, #7573, #6956, #7663, #1580, #3004, #4145, #4981, #4316, #5022, #5546, #7615, #6171, #2873, #963, #8382, #4933, #7000, #6823, #5587, #4273, #787, #4895, #2826, #1490, #3575, #301, #4228, #215, #8251, #5498, #3489, #256, #5634, #127, #2210, #8208 ) ),
 .UNSPECIFIED., .F., .F., .T. ) 
 B_SPLINE_SURFACE_WITH_KNOTS ( ( 2, 1, 2 ),
 ( 3, 2, 2, 2, 2, 2, 2, 2, 2, 2, 2, 2, 2, 2, 2, 2, 2, 2, 2, 2, 2, 2, 2, 2, 2, 2, 2, 2, 2, 2, 2, 2, 2, 2, 2, 2, 2, 2, 2, 2, 2, 2, 2, 2, 2, 2, 2, 2, 2, 2, 2, 2, 3 ),
 ( -0.01000000000000000021, 0.000000000000000000, 1.000000000000000000 ),
 ( -0.008928571428571429811, 0.000000000000000000, 0.01785714285714285615, 0.03571428571428571230, 0.05357142857142856845, 0.07142857142857142461, 0.08928571428571428770, 0.1071428571428571369, 0.1250000000000000000, 0.1428571428571428492, 0.1607142857142857262, 0.1785714285714285754, 0.1964285714285714246, 0.2142857142857142738, 0.2321428571428571508, 0.2500000000000000000, 0.2678571428571428492, 0.2857142857142856984, 0.3035714285714285476, 0.3214285714285714524, 0.3392857142857143016, 0.3571428571428571508, 0.3750000000000000000, 0.3928571428571428492, 0.4107142857142856984, 0.4285714285714285476, 0.4464285714285714524, 0.4642857142857143016, 0.4821428571428571508, 0.5000000000000000000, 0.5178571428571429047, 0.5357142857142856984, 0.5535714285714286031, 0.5714285714285713969, 0.5892857142857143016, 0.6071428571428570953, 0.6250000000000000000, 0.6428571428571429047, 0.6607142857142856984, 0.6785714285714286031, 0.6964285714285713969, 0.7142857142857143016, 0.7321428571428570953, 0.7500000000000000000, 0.7678571428571429047, 0.7857142857142856984, 0.8035714285714286031, 0.8214285714285713969, 0.8392857142857143016, 0.8571428571428570953, 0.8750000000000000000, 0.8928571428571429047, 0.9018750000000000933 ),
 .UNSPECIFIED. ) 
 GEOMETRIC_REPRESENTATION_ITEM ( )  RATIONAL_B_SPLINE_SURFACE ( (
 ( 1.000000000000000000, 1.000000000000000000, 1.000000000000000000, 0.9238795325112867385, 1.000000000000000000, 0.9238795325112867385, 1.000000000000000000, 0.9238795325112867385, 1.000000000000000000, 0.9238795325112867385, 1.000000000000000000, 0.9238795325112867385, 1.000000000000000000, 0.9238795325112867385, 1.000000000000000000, 0.9238795325112867385, 1.000000000000000000, 0.9238795325112867385, 1.000000000000000000, 0.9238795325112867385, 1.000000000000000000, 0.9238795325112867385, 1.000000000000000000, 0.9238795325112867385, 1.000000000000000000, 0.9238795325112867385, 1.000000000000000000, 0.9238795325112867385, 1.000000000000000000, 0.9238795325112867385, 1.000000000000000000, 0.9238795325112867385, 1.000000000000000000, 0.9238795325112867385, 1.000000000000000000, 0.9238795325112867385, 1.000000000000000000, 0.9238795325112867385, 1.000000000000000000, 0.9238795325112867385, 1.000000000000000000, 0.9238795325112867385, 1.000000000000000000, 0.9238795325112867385, 1.000000000000000000, 0.9238795325112867385, 1.000000000000000000, 0.9238795325112867385, 1.000000000000000000, 0.9238795325112867385, 1.000000000000000000, 0.9238795325112867385, 1.000000000000000000, 0.9238795325112867385, 1.000000000000000000, 0.9238795325112867385, 1.000000000000000000, 0.9238795325112867385, 1.000000000000000000, 0.9238795325112867385, 1.000000000000000000, 0.9238795325112867385, 1.000000000000000000, 0.9238795325112867385, 1.000000000000000000, 0.9238795325112867385, 1.000000000000000000, 0.9238795325112867385, 1.000000000000000000, 0.9238795325112867385, 1.000000000000000000, 0.9238795325112867385, 1.000000000000000000, 0.9238795325112867385, 1.000000000000000000, 0.9238795325112867385, 1.000000000000000000, 0.9238795325112867385, 1.000000000000000000, 0.9238795325112867385, 1.000000000000000000, 0.9238795325112867385, 1.000000000000000000, 0.9238795325112867385, 1.000000000000000000, 0.9238795325112867385, 1.000000000000000000, 0.9238795325112867385, 1.000000000000000000, 0.9238795325112867385, 1.000000000000000000, 0.9238795325112867385, 1.000000000000000000, 0.9238795325112867385, 1.000000000000000000, 0.9238795325112867385, 1.000000000000000000, 0.9238795325112867385, 1.000000000000000000, 0.9238795325112867385, 1.000000000000000000, 0.9238795325112867385, 1.000000000000000000, 1.000000000000000000, 1.000000000000000000),
 ( 1.000000000000000000, 1.000000000000000000, 1.000000000000000000, 0.9238795325112867385, 1.000000000000000000, 0.9238795325112867385, 1.000000000000000000, 0.9238795325112867385, 1.000000000000000000, 0.9238795325112867385, 1.000000000000000000, 0.9238795325112867385, 1.000000000000000000, 0.9238795325112867385, 1.000000000000000000, 0.9238795325112867385, 1.000000000000000000, 0.9238795325112867385, 1.000000000000000000, 0.9238795325112867385, 1.000000000000000000, 0.9238795325112867385, 1.000000000000000000, 0.9238795325112867385, 1.000000000000000000, 0.9238795325112867385, 1.000000000000000000, 0.9238795325112867385, 1.000000000000000000, 0.9238795325112867385, 1.000000000000000000, 0.9238795325112867385, 1.000000000000000000, 0.9238795325112867385, 1.000000000000000000, 0.9238795325112867385, 1.000000000000000000, 0.9238795325112867385, 1.000000000000000000, 0.9238795325112867385, 1.000000000000000000, 0.9238795325112867385, 1.000000000000000000, 0.9238795325112867385, 1.000000000000000000, 0.9238795325112867385, 1.000000000000000000, 0.9238795325112867385, 1.000000000000000000, 0.9238795325112867385, 1.000000000000000000, 0.9238795325112867385, 1.000000000000000000, 0.9238795325112867385, 1.000000000000000000, 0.9238795325112867385, 1.000000000000000000, 0.9238795325112867385, 1.000000000000000000, 0.9238795325112867385, 1.000000000000000000, 0.9238795325112867385, 1.000000000000000000, 0.9238795325112867385, 1.000000000000000000, 0.9238795325112867385, 1.000000000000000000, 0.9238795325112867385, 1.000000000000000000, 0.9238795325112867385, 1.000000000000000000, 0.9238795325112867385, 1.000000000000000000, 0.9238795325112867385, 1.000000000000000000, 0.9238795325112867385, 1.000000000000000000, 0.9238795325112867385, 1.000000000000000000, 0.9238795325112867385, 1.000000000000000000, 0.9238795325112867385, 1.000000000000000000, 0.9238795325112867385, 1.000000000000000000, 0.9238795325112867385, 1.000000000000000000, 0.9238795325112867385, 1.000000000000000000, 0.9238795325112867385, 1.000000000000000000, 0.9238795325112867385, 1.000000000000000000, 0.9238795325112867385, 1.000000000000000000, 0.9238795325112867385, 1.000000000000000000, 0.9238795325112867385, 1.000000000000000000, 0.9238795325112867385, 1.000000000000000000, 0.9238795325112867385, 1.000000000000000000, 1.000000000000000000, 1.000000000000000000),
 ( 1.000000000000000000, 1.000000000000000000, 1.000000000000000000, 0.9238795325112867385, 1.000000000000000000, 0.9238795325112867385, 1.000000000000000000, 0.9238795325112867385, 1.000000000000000000, 0.9238795325112867385, 1.000000000000000000, 0.9238795325112867385, 1.000000000000000000, 0.9238795325112867385, 1.000000000000000000, 0.9238795325112867385, 1.000000000000000000, 0.9238795325112867385, 1.000000000000000000, 0.9238795325112867385, 1.000000000000000000, 0.9238795325112867385, 1.000000000000000000, 0.9238795325112867385, 1.000000000000000000, 0.9238795325112867385, 1.000000000000000000, 0.9238795325112867385, 1.000000000000000000, 0.9238795325112867385, 1.000000000000000000, 0.9238795325112867385, 1.000000000000000000, 0.9238795325112867385, 1.000000000000000000, 0.9238795325112867385, 1.000000000000000000, 0.9238795325112867385, 1.000000000000000000, 0.9238795325112867385, 1.000000000000000000, 0.9238795325112867385, 1.000000000000000000, 0.9238795325112867385, 1.000000000000000000, 0.9238795325112867385, 1.000000000000000000, 0.9238795325112867385, 1.000000000000000000, 0.9238795325112867385, 1.000000000000000000, 0.9238795325112867385, 1.000000000000000000, 0.9238795325112867385, 1.000000000000000000, 0.9238795325112867385, 1.000000000000000000, 0.9238795325112867385, 1.000000000000000000, 0.9238795325112867385, 1.000000000000000000, 0.9238795325112867385, 1.000000000000000000, 0.9238795325112867385, 1.000000000000000000, 0.9238795325112867385, 1.000000000000000000, 0.9238795325112867385, 1.000000000000000000, 0.9238795325112867385, 1.000000000000000000, 0.9238795325112867385, 1.000000000000000000, 0.9238795325112867385, 1.000000000000000000, 0.9238795325112867385, 1.000000000000000000, 0.9238795325112867385, 1.000000000000000000, 0.9238795325112867385, 1.000000000000000000, 0.9238795325112867385, 1.000000000000000000, 0.9238795325112867385, 1.000000000000000000, 0.9238795325112867385, 1.000000000000000000, 0.9238795325112867385, 1.000000000000000000, 0.9238795325112867385, 1.000000000000000000, 0.9238795325112867385, 1.000000000000000000, 0.9238795325112867385, 1.000000000000000000, 0.9238795325112867385, 1.000000000000000000, 0.9238795325112867385, 1.000000000000000000, 0.9238795325112867385, 1.000000000000000000, 0.9238795325112867385, 1.000000000000000000, 1.000000000000000000, 1.000000000000000000) ) ) 
 REPRESENTATION_ITEM ( '' )  SURFACE ( )  );
#6423=FACE_OUTER_BOUND ( 'NONE', #2393, .T. ) ;
#6428=CARTESIAN_POINT ( 'NONE',  ( 2.071067811865477282, -49.99999999999996447, -95.54999999999999716 ) ) ;
#6435=CARTESIAN_POINT ( 'NONE',  ( -3.061616997868382155E-16, -39.99999999999997158, -98.40000000000000568 ) ) ;
#6436=CARTESIAN_POINT ( 'NONE',  ( -4.999999999999998224, -44.99999999999997158, -98.09999999781504698 ) ) ;
#6442=CARTESIAN_POINT ( 'NONE',  ( 4.999999999999998224, -44.99999999999997158, -98.60000000000000853 ) ) ;
#6451=CARTESIAN_POINT ( 'NONE',  ( -2.796473189345805913E-16, -40.43301269999997061, -100.2499999989075263 ) ) ;
#6455=CARTESIAN_POINT ( 'NONE',  ( -4.566987299999997418, -46.89170807884566727, -96.19999999890751496 ) ) ;
#6463=CARTESIAN_POINT ( 'NONE',  ( -3.061616997868382155E-16, -39.99999999999997158, -96.69999999781504130 ) ) ;
#6465=CARTESIAN_POINT ( 'NONE',  ( 3.535533905932736420, -41.46446609406723383, -97.59999999781504698 ) ) ;
#6466=LINE ( 'NONE', #3005, #2858 ) ;
#6467=CARTESIAN_POINT ( 'NONE',  ( 3.535533905932737309, -48.53553390593270933, -97.10000000000000853 ) ) ;
#6471=SHAPE_REPRESENTATION ( 'position indicator', ( #2554 ), #564 ) ;
#6473=CARTESIAN_POINT ( 'NONE',  ( -2.071067811865475061, -39.99999999999997158, -99.14999999999999147 ) ) ;
#6475=CARTESIAN_POINT ( 'NONE',  ( -2.449416140927843877, -49.39737961008592038, -100.0005770061920884 ) ) ;
#6477=CYLINDRICAL_SURFACE ( 'NONE', #7074, 4.999999999999998224 ) ;
#6481=DIRECTION ( 'NONE',  ( -1.000000000000000000, 0.000000000000000000, 0.000000000000000000 ) ) ;
#6491=CARTESIAN_POINT ( 'NONE',  ( -4.566987299999997418, -46.89170807884566017, -99.99999999890754054 ) ) ;
#6495=CARTESIAN_POINT ( 'NONE',  ( 8.389419568037416259E-16, -49.56698729999997255, -100.0499999989075093 ) ) ;
#6497=CARTESIAN_POINT ( 'NONE',  ( -3.229347689422839451, -48.22934768942280925, -96.94999999890751496 ) ) ;
#6505=FACE_OUTER_BOUND ( 'NONE', #3997, .T. ) ;
#6509=CARTESIAN_POINT ( 'NONE',  ( -4.999999999999998224, -44.99999999999997158, -97.40000000000000568 ) ) ;
#6515=CARTESIAN_POINT ( 'NONE',  ( -3.535533905932736864, -41.46446609406723383, -97.50000000000000000 ) ) ;
#6517=CARTESIAN_POINT ( 'NONE',  ( 0.3202549665280822189, -49.99785177082193854, -100.0005802109309059 ) ) ;
#6526=CARTESIAN_POINT ( 'NONE',  ( 0.000000000000000000, -44.99999999999997158, -95.00000000000000000 ) ) ;
#6533=CARTESIAN_POINT ( 'NONE',  ( 4.566987299999998307, -43.10829192115428299, -98.79999999890750928 ) ) ;
#6537=CARTESIAN_POINT ( 'NONE',  ( -4.566987299999998307, -44.99999999999997158, -100.2499999989075121 ) ) ;
#6539=CARTESIAN_POINT ( 'NONE',  ( 4.566987299999998307, -43.10829192115428299, -96.39999999890753202 ) ) ;
#6551=LINE ( 'NONE', #593, #1870 ) ;
#6552=CARTESIAN_POINT ( 'NONE',  ( 4.999999999999998224, -44.99999999999997158, -99.40000000000000568 ) ) ;
#6559=CARTESIAN_POINT ( 'NONE',  ( 2.071067811865474173, -39.99999999999997158, -96.85000000000002274 ) ) ;
#6562=CARTESIAN_POINT ( 'NONE',  ( -3.397431688313778952, -41.32060051903346931, -99.99956440458885254 ) ) ;
#6580=CARTESIAN_POINT ( 'NONE',  ( 1.891708078845682595, -40.43301269999998482, -96.29999999890752349 ) ) ;
#6586=VERTEX_POINT ( 'NONE', #5853 ) ;
#6592=CARTESIAN_POINT ( 'NONE',  ( -4.999999999999998224, -44.99999999999997158, -96.60000000000000853 ) ) ;
#6594=ORIENTED_EDGE ( 'NONE', *, *, #5517, .F. ) ;
#6599=CARTESIAN_POINT ( 'NONE',  ( 4.999999999999998224, -42.92893218813448897, -96.84999999781504698 ) ) ;
#6601=CARTESIAN_POINT ( 'NONE',  ( 1.891708078845685481, -49.56698729999997255, -99.79999999890752349 ) ) ;
#6602=CARTESIAN_POINT ( 'NONE',  ( -5.005283159123838921, -45.16039493131476235, -100.0002415582530517 ) ) ;
#6604=AXIS2_PLACEMENT_3D ( 'NONE', #2002, #3942, #8139 ) ;
#6605=CARTESIAN_POINT ( 'NONE',  ( -4.999999999999998224, -42.92893218813448897, -95.84300000002187403 ) ) ;
#6621=CARTESIAN_POINT ( 'NONE',  ( -1.891708078845683039, -40.43301269999998482, -98.79999999890753770 ) ) ;
#6624=DIRECTION ( 'NONE',  ( -0.000000000000000000, -0.000000000000000000, 1.000000000000000000 ) ) ;
#6633=CARTESIAN_POINT ( 'NONE',  ( 4.999999999999998224, -44.99999999999997158, -99.29999999781504982 ) ) ;
#6636=CARTESIAN_POINT ( 'NONE',  ( 2.071067811865474173, -39.99999999999997158, -99.25000000000000000 ) ) ;
#6642=CARTESIAN_POINT ( 'NONE',  ( -4.566987299999998307, -43.10829192115428299, -98.69999999890752918 ) ) ;
#6643=CARTESIAN_POINT ( 'NONE',  ( -4.999999999999998224, -42.92893218813448897, -99.85000000000002274 ) ) ;
#6645=CARTESIAN_POINT ( 'NONE',  ( 4.566987299999998307, -43.10829192115428299, -97.19999999890752918 ) ) ;
#6647=CARTESIAN_POINT ( 'NONE',  ( -4.991843310627483099, -44.59989201564595618, -99.99932436085771315 ) ) ;
#6652=CARTESIAN_POINT ( 'NONE',  ( 9.184850993605145972E-16, -49.99999999999997158, -97.19300000002183992 ) ) ;
#6664=CARTESIAN_POINT ( 'NONE',  ( 4.999999999999998224, -44.99999999999997158, -97.00000000000000000 ) ) ;
#6667=CARTESIAN_POINT ( 'NONE',  ( -2.071067811865475061, -39.99999999999997158, -99.04999999781504982 ) ) ;
#6669=CARTESIAN_POINT ( 'NONE',  ( 3.229347689422839895, -41.77065231057713390, -95.54999999890752349 ) ) ;
#6677=VERTEX_POINT ( 'NONE', #2389 ) ;
#6681=CARTESIAN_POINT ( 'NONE',  ( -3.229347689422840784, -41.77065231057713390, -95.54999999890752349 ) ) ;
#6682=DIRECTION ( 'NONE',  ( -0.000000000000000000, -0.000000000000000000, -1.000000000000000000 ) ) ;
#6683=CARTESIAN_POINT ( 'NONE',  ( -2.071067811865475505, -49.99999999999996447, -98.04999999999999716 ) ) ;
#6689=CARTESIAN_POINT ( 'NONE',  ( 4.566987299999998307, -43.10829192115428299, -98.19999999890752918 ) ) ;
#6690=CARTESIAN_POINT ( 'NONE',  ( -2.071067811865475061, -39.99999999999997158, -97.44999999781505551 ) ) ;
#6692=CARTESIAN_POINT ( 'NONE',  ( -1.891708078845683483, -49.56698729999997255, -98.29999999890752349 ) ) ;
#6693=PRESENTATION_STYLE_ASSIGNMENT (( #2032 ) ) ;
#6695=CARTESIAN_POINT ( 'NONE',  ( -2.071067811865475061, -39.99999999999997158, -96.74300000002187971 ) ) ;
#6696=( BOUNDED_CURVE ( )  B_SPLINE_CURVE ( 2, ( #5430, #13, #4248, #5521, #2713, #8269, #8140, #3510, #5383 ),
 .UNSPECIFIED., .F., .T. ) 
 B_SPLINE_CURVE_WITH_KNOTS ( ( 3, 2, 2, 2, 3 ),
 ( 0.6428571428571429047, 0.6607142857142856984, 0.6785714285714286031, 0.6964285714285713969, 0.7142857142857143016 ),
 .UNSPECIFIED. ) 
 CURVE ( )  GEOMETRIC_REPRESENTATION_ITEM ( )  RATIONAL_B_SPLINE_CURVE ( ( 1.000000000000000000, 0.9238795325112867385, 1.000000000000000000, 0.9238795325112867385, 1.000000000000000000, 0.9238795325112867385, 1.000000000000000000, 0.9238795325112867385, 1.000000000000000000 ) ) 
 REPRESENTATION_ITEM ( '' )  );
#6702=CARTESIAN_POINT ( 'NONE',  ( 9.184850993605145972E-16, -49.99999999999997158, -99.59999999999999432 ) ) ;
#6712=CARTESIAN_POINT ( 'NONE',  ( -2.796473189345805913E-16, -40.43301269999997061, -99.64999999890751781 ) ) ;
#6720=ORIENTED_EDGE ( 'NONE', *, *, #2327, .F. ) ;
#6726=CARTESIAN_POINT ( 'NONE',  ( -4.999999999999998224, -42.92893218813448897, -100.5499999978150498 ) ) ;
#6730=ORIENTED_EDGE ( 'NONE', *, *, #2970, .T. ) ;
#6734=CARTESIAN_POINT ( 'NONE',  ( -4.566987299999998307, -44.99999999999997158, -96.24999999890751212 ) ) ;
#6735=CARTESIAN_POINT ( 'NONE',  ( -2.071067811865475505, -49.99999999999996447, -96.34999999781506119 ) ) ;
#6737=CARTESIAN_POINT ( 'NONE',  ( -2.796473189345805913E-16, -40.43301269999997061, -99.44999999890752918 ) ) ;
#6738=FACE_BOUND ( 'NONE', #8621, .T. ) ;
#6740=CARTESIAN_POINT ( 'NONE',  ( 3.535533905932737309, -48.53553390593270933, -95.49300000002185129 ) ) ;
#6752=PLANE ( 'NONE',  #6604 ) ;
#6755=CARTESIAN_POINT ( 'NONE',  ( 3.535533905932737309, -48.53553390593270933, -98.70000000000000284 ) ) ;
#6761=ORIENTED_EDGE ( 'NONE', *, *, #8716, .F. ) ;
#6765=CARTESIAN_POINT ( 'NONE',  ( -3.061616997868382155E-16, -39.99999999999997158, -99.89999999781504414 ) ) ;
#6767=CARTESIAN_POINT ( 'NONE',  ( -3.535533905932735532, -48.53553390593270933, -96.39999999781505835 ) ) ;
#6772=VERTEX_POINT ( 'NONE', #4577 ) ;
#6773=EDGE_CURVE ( 'NONE', #2955, #5525, #6551, .T. ) ;
#6775=CARTESIAN_POINT ( 'NONE',  ( 4.566987299999998307, -44.99999999999997158, -97.44999999890751496 ) ) ;
#6776=CARTESIAN_POINT ( 'NONE',  ( 1.932551333443697450, -39.99999999999997158, -100.0466559163918419 ) ) ;
#6778=CARTESIAN_POINT ( 'NONE',  ( 1.891708078845682595, -40.43301269999998482, -97.09999999890753486 ) ) ;
#6783=CARTESIAN_POINT ( 'NONE',  ( 5.000000000000000000, -47.07106781186545419, -96.24300000002185129 ) ) ;
#6788=EDGE_CURVE ( 'NONE', #2418, #5152, #4906, .T. ) ;
#6797=CARTESIAN_POINT ( 'NONE',  ( -4.566987299999998307, -44.99999999999997158, -95.44999999890751496 ) ) ;
#6814=CARTESIAN_POINT ( 'NONE',  ( -4.999999999999998224, -42.92893218813448897, -98.94999999781504130 ) ) ;
#6822=CARTESIAN_POINT ( 'NONE',  ( 8.389419568037416259E-16, -49.56698729999997255, -98.44999999890752918 ) ) ;
#6823=CARTESIAN_POINT ( 'NONE',  ( -3.061616997868382155E-16, -39.99999999999997158, -99.89999999781504414 ) ) ;
#6825=CARTESIAN_POINT ( 'NONE',  ( 4.566987300000000083, -46.89170807884565306, -98.09999999890752065 ) ) ;
#6826=( NAMED_UNIT ( * ) SI_UNIT ( $, .STERADIAN. ) SOLID_ANGLE_UNIT ( ) );
#6828=CARTESIAN_POINT ( 'NONE',  ( -3.535533905932736864, -41.46446609406723383, -99.09300000002185982 ) ) ;
#6853=CARTESIAN_POINT ( 'NONE',  ( -3.229347689422840784, -41.77065231057713390, -96.94999999890751496 ) ) ;
#6856=CARTESIAN_POINT ( 'NONE',  ( -4.566987299999997418, -46.89170807884566727, -96.99999999890751212 ) ) ;
#6863=ORIENTED_EDGE ( 'NONE', *, *, #1726, .F. ) ;
#6865=CARTESIAN_POINT ( 'NONE',  ( 0.000000000000000000, -44.99999999999997158, -95.00000000000000000 ) ) ;
#6866=CARTESIAN_POINT ( 'NONE',  ( -2.796473189345805913E-16, -40.43301269999997061, -99.64999999890751781 ) ) ;
#6869=CARTESIAN_POINT ( 'NONE',  ( 1.891708078845682595, -40.43301269999998482, -97.89999999890753202 ) ) ;
#6873=CARTESIAN_POINT ( 'NONE',  ( 2.071067811865474173, -39.99999999999997158, -96.04999999999999716 ) ) ;
#6874=CARTESIAN_POINT ( 'NONE',  ( 3.229347689422839895, -41.77065231057713390, -96.34999999890753486 ) ) ;
#6876=CARTESIAN_POINT ( 'NONE',  ( 3.535533905932736420, -41.46446609406723383, -95.99999999781503845 ) ) ;
#6885=DIRECTION ( 'NONE',  ( -1.000000000000000000, 0.000000000000000000, 0.000000000000000000 ) ) ;
#6895=ORIENTED_EDGE ( 'NONE', *, *, #1709, .T. ) ;
#6896=CARTESIAN_POINT ( 'NONE',  ( -3.229347689422840784, -41.77065231057713390, -95.34999999890753486 ) ) ;
#6898=FACE_OUTER_BOUND ( 'NONE', #8313, .T. ) ;
#6900=CARTESIAN_POINT ( 'NONE',  ( -3.229347689422839451, -48.22934768942280925, -96.94999999890751496 ) ) ;
#6910=CARTESIAN_POINT ( 'NONE',  ( 1.891708078845682595, -40.43301269999998482, -99.69999999890752918 ) ) ;
#6913=CARTESIAN_POINT ( 'NONE',  ( 4.566987300000000083, -46.89170807884565306, -99.69999999890752918 ) ) ;
#6916=CARTESIAN_POINT ( 'NONE',  ( -3.535533905932736864, -41.46446609406723383, -95.90000000000000568 ) ) ;
#6922=SHAPE_DEFINITION_REPRESENTATION ( #2973, #6471 ) ;
#6929=CARTESIAN_POINT ( 'NONE',  ( 4.999999999999998224, -44.99999999999997158, -97.79999999999999716 ) ) ;
#6940=EDGE_CURVE ( 'NONE', #5592, #2848, #7608, .T. ) ;
#6941=CARTESIAN_POINT ( 'NONE',  ( -3.229347689422839451, -48.22934768942280925, -96.74999999890752633 ) ) ;
#6943=CYLINDRICAL_SURFACE ( 'NONE', #2927, 4.999999999999998224 ) ;
#6944=CARTESIAN_POINT ( 'NONE',  ( 1.891708078845682595, -40.43301269999998482, -98.09999999890750644 ) ) ;
#6946=DIRECTION ( 'NONE',  ( -1.000000000000000000, 0.000000000000000000, 0.000000000000000000 ) ) ;
#6954=CARTESIAN_POINT ( 'NONE',  ( -1.891708078845683705, -49.56698729999997255, -100.0999999989075206 ) ) ;
#6956=CARTESIAN_POINT ( 'NONE',  ( -3.061616997868382155E-16, -39.99999999999997158, -99.09999999781504698 ) ) ;
#6957=DIRECTION ( 'NONE',  ( -1.000000000000000000, 0.000000000000000000, 0.000000000000000000 ) ) ;
#6958=CARTESIAN_POINT ( 'NONE',  ( 4.566987299999998307, -43.10829192115428299, -98.79999999890753770 ) ) ;
#6959=ORIENTED_EDGE ( 'NONE', *, *, #4668, .T. ) ;
#6962=CARTESIAN_POINT ( 'NONE',  ( -3.535533905932735532, -48.53553390593270933, -99.69300000002185413 ) ) ;
#6963=CARTESIAN_POINT ( 'NONE',  ( -4.566987299999998307, -44.99999999999997158, -95.24999999890752633 ) ) ;
#6971=CARTESIAN_POINT ( 'NONE',  ( 4.999999999999998224, -42.92893218813449607, -98.54999999999999716 ) ) ;
#6973=CARTESIAN_POINT ( 'NONE',  ( 3.072733599874575727, -41.00166578800908468, -100.0000000000000142 ) ) ;
#6975=ORIENTED_EDGE ( 'NONE', *, *, #8464, .F. ) ;
#6977=ORIENTED_EDGE ( 'NONE', *, *, #4037, .F. ) ;
#6984=CARTESIAN_POINT ( 'NONE',  ( -2.796473189345805913E-16, -40.43301269999997061, -96.24999999890752633 ) ) ;
#6987=CARTESIAN_POINT ( 'NONE',  ( 3.229347689422841228, -48.22934768942280925, -97.54999999890752349 ) ) ;
#6989=CARTESIAN_POINT ( 'NONE',  ( 1.891708078845685481, -49.56698729999997255, -98.39999999890753202 ) ) ;
#6991=ORIENTED_EDGE ( 'NONE', *, *, #6940, .T. ) ;
#6997=DIRECTION ( 'NONE',  ( -0.000000000000000000, -0.000000000000000000, -1.000000000000000000 ) ) ;
#7000=CARTESIAN_POINT ( 'NONE',  ( -2.071067811865475061, -39.99999999999997158, -99.84999999781504698 ) ) ;
#7003=CARTESIAN_POINT ( 'NONE',  ( -3.229347689422840784, -41.77065231057713390, -98.54999999890752349 ) ) ;
#7006=AXIS2_PLACEMENT_3D ( 'NONE', #5105, #1763, #5020 ) ;
#7007=CARTESIAN_POINT ( 'NONE',  ( -3.535533905932735532, -48.53553390593270933, -98.89300000002185698 ) ) ;
#7009=CARTESIAN_POINT ( 'NONE',  ( 4.999999999999998224, -42.92893218813448897, -97.64999999781504414 ) ) ;
#7011=CARTESIAN_POINT ( 'NONE',  ( -3.061616997868382155E-16, -39.99999999999997158, -100.6999999978150555 ) ) ;
#7027=CARTESIAN_POINT ( 'NONE',  ( -4.566987299999998307, -43.10829192115428299, -100.0999999989075349 ) ) ;
#7030=CARTESIAN_POINT ( 'NONE',  ( 8.389419568037416259E-16, -49.56698729999997255, -98.44999999890752918 ) ) ;
#7032=CARTESIAN_POINT ( 'NONE',  ( -4.566987299999998307, -44.99999999999997158, -97.84999999890752065 ) ) ;
#7041=( BOUNDED_CURVE ( )  B_SPLINE_CURVE ( 2, ( #4300, #8238, #5573, #1521, #8321 ),
 .UNSPECIFIED., .F., .T. ) 
 B_SPLINE_CURVE_WITH_KNOTS ( ( 3, 2, 3 ),
 ( 0.8571428571428572063, 0.8750000000000000000, 0.8928571428571429047 ),
 .UNSPECIFIED. ) 
 CURVE ( )  GEOMETRIC_REPRESENTATION_ITEM ( )  RATIONAL_B_SPLINE_CURVE ( ( 0.9999999999999995559, 0.9238795325112871826, 1.000000000000000000, 0.9238795325112867385, 1.000000000000000000 ) ) 
 REPRESENTATION_ITEM ( '' )  );
#7042=CARTESIAN_POINT ( 'NONE',  ( 4.999999999999998224, -44.99999999999997158, -96.89999999781505835 ) ) ;
#7043=CARTESIAN_POINT ( 'NONE',  ( 4.999999999999998224, -44.99999999999997158, -98.49999999781503845 ) ) ;
#7044=DIRECTION ( 'NONE',  ( 6.123233995736960786E-17, -1.000000000000000000, 0.000000000000000000 ) ) ;
#7047=CARTESIAN_POINT ( 'NONE',  ( 3.535533905932736420, -41.46446609406723383, -96.10000000000000853 ) ) ;
#7053=ORIENTED_EDGE ( 'NONE', *, *, #257, .F. ) ;
#7054=CARTESIAN_POINT ( 'NONE',  ( -3.229347689422840784, -41.77065231057713390, -95.34999999890753486 ) ) ;
#7055=CARTESIAN_POINT ( 'NONE',  ( -4.999999999999998224, -42.92893218813448897, -95.74999999781503845 ) ) ;
#7061=CARTESIAN_POINT ( 'NONE',  ( 1.891708078845682595, -40.43301269999998482, -95.69999999890751496 ) ) ;
#7062=PRODUCT_DEFINITION_FORMATION_WITH_SPECIFIED_SOURCE ( 'ANY', '', #3671, .NOT_KNOWN. ) ;
#7074=AXIS2_PLACEMENT_3D ( 'NONE', #4458, #7352, #5690 ) ;
#7076=LINE ( 'NONE', #1035, #8411 ) ;
#7083=CARTESIAN_POINT ( 'NONE',  ( 4.566987300000000083, -46.89170807884565306, -95.89999999890753202 ) ) ;
#7094=CARTESIAN_POINT ( 'NONE',  ( -3.535533905932736864, -41.46446609406723383, -95.10000000000000853 ) ) ;
#7099=ORIENTED_EDGE ( 'NONE', *, *, #6388, .T. ) ;
#7100=CARTESIAN_POINT ( 'NONE',  ( -2.071067811865475061, -39.99999999999997158, -97.54999999999998295 ) ) ;
#7101=CARTESIAN_POINT ( 'NONE',  ( -2.071067811865475505, -49.99999999999996447, -97.94999999781504130 ) ) ;
#7105=CARTESIAN_POINT ( 'NONE',  ( -4.999999999999998224, -44.99999999999997158, -99.69999999781505551 ) ) ;
#7114=CIRCLE ( 'NONE', #782, 4.999999999999998224 ) ;
#7115=CARTESIAN_POINT ( 'NONE',  ( 4.566987299999998307, -44.99999999999997158, -99.64999999890753202 ) ) ;
#7120=CARTESIAN_POINT ( 'NONE',  ( 8.389419568037416259E-16, -49.56698729999997255, -96.04999999890752349 ) ) ;
#7128=CYLINDRICAL_SURFACE ( 'NONE', #6011, 7.499999999999999112 ) ;
#7130=CARTESIAN_POINT ( 'NONE',  ( 4.999999999999996447, -47.07106781186543998, -95.45000000000000284 ) ) ;
#7133=CARTESIAN_POINT ( 'NONE',  ( 3.535533905932736420, -41.46446609406723383, -96.90000000000000568 ) ) ;
#7137=ORIENTED_EDGE ( 'NONE', *, *, #5864, .F. ) ;
#7139=CARTESIAN_POINT ( 'NONE',  ( 3.535533905932736420, -41.46446609406723383, -98.50000000000000000 ) ) ;
#7141=FACE_OUTER_BOUND ( 'NONE', #33, .T. ) ;
#7142=CARTESIAN_POINT ( 'NONE',  ( 0.8856097000871558933, -49.92917650584813316, -100.0008279209158388 ) ) ;
#7144=EDGE_CURVE ( 'NONE', #1056, #5746, #4004, .T. ) ;
#7146=CARTESIAN_POINT ( 'NONE',  ( -4.999999999999998224, -44.99999999999997158, -98.19999999999998863 ) ) ;
#7156=CARTESIAN_POINT ( 'NONE',  ( 3.229347689422841228, -48.22934768942280925, -99.74999999890752633 ) ) ;
#7162=CARTESIAN_POINT ( 'NONE',  ( 4.566987299999998307, -43.10829192115428299, -95.79999999890752349 ) ) ;
#7165=CARTESIAN_POINT ( 'NONE',  ( -4.999999999999998224, -44.99999999999997158, -95.00000000000000000 ) ) ;
#7174=CARTESIAN_POINT ( 'NONE',  ( -4.999999999999997335, -47.07106781186546129, -97.35000000000000853 ) ) ;
#7182=CARTESIAN_POINT ( 'NONE',  ( -3.535533905932736864, -41.46446609406723383, -98.29999999999999716 ) ) ;
#7183=CARTESIAN_POINT ( 'NONE',  ( 4.712883770844864983, -46.76680472316598980, -99.99969226647576193 ) ) ;
#7193=ORIENTED_EDGE ( 'NONE', *, *, #6394, .F. ) ;
#7198=CARTESIAN_POINT ( 'NONE',  ( 3.535533905932736420, -41.46446609406723383, -96.10000000000000853 ) ) ;
#7204=CARTESIAN_POINT ( 'NONE',  ( 8.389419568037416259E-16, -49.56698729999997255, -99.24999999890751212 ) ) ;
#7216=FACE_OUTER_BOUND ( 'NONE', #3722, .T. ) ;
#7218=CARTESIAN_POINT ( 'NONE',  ( 4.999999999999998224, -42.92893218813448897, -96.15000000000000568 ) ) ;
#7223=CARTESIAN_POINT ( 'NONE',  ( -4.999999999999997335, -47.07106781186546129, -98.95000000000000284 ) ) ;
#7225=CARTESIAN_POINT ( 'NONE',  ( 1.999693926619486195, -49.61910733158132558, -99.99999752325564373 ) ) ;
#7226=EDGE_CURVE ( 'NONE', #5746, #7878, #2455, .T. ) ;
#7230=CARTESIAN_POINT ( 'NONE',  ( -4.999999999999998224, -44.99999999999997158, -97.29999999781504982 ) ) ;
#7246=CARTESIAN_POINT ( 'NONE',  ( -1.891708078845683483, -49.56698729999997255, -95.89999999890753202 ) ) ;
#7259=CARTESIAN_POINT ( 'NONE',  ( -3.061616997868382155E-16, -39.99999999999997158, -98.40000000000000568 ) ) ;
#7266=CARTESIAN_POINT ( 'NONE',  ( 4.999999999999998224, -42.92893218813448897, -96.95000000000000284 ) ) ;
#7268=CARTESIAN_POINT ( 'NONE',  ( 8.389419568037416259E-16, -49.56698729999997255, -99.04999999890752349 ) ) ;
#7273=CARTESIAN_POINT ( 'NONE',  ( 2.071067811865474173, -39.99999999999997158, -96.04300000002184845 ) ) ;
#7283=CARTESIAN_POINT ( 'NONE',  ( 3.535533905932736420, -41.46446609406723383, -96.90000000000000568 ) ) ;
#7287=EDGE_CURVE ( 'NONE', #5592, #196, #2332, .T. ) ;
#7290=CARTESIAN_POINT ( 'NONE',  ( -1.891708078845683483, -49.56698729999997255, -100.0999999989075206 ) ) ;
#7301=CARTESIAN_POINT ( 'NONE',  ( -2.071067811865475061, -39.99999999999997158, -100.6499999978150441 ) ) ;
#7309=CARTESIAN_POINT ( 'NONE',  ( 2.071067811865474173, -39.99999999999997158, -95.94999999781504130 ) ) ;
#7311=CARTESIAN_POINT ( 'NONE',  ( -1.891708078845683039, -40.43301269999998482, -99.39999999890751781 ) ) ;
#7317=CARTESIAN_POINT ( 'NONE',  ( 4.999999999999998224, -42.92893218813448897, -95.34300000002184561 ) ) ;
#7319=( BOUNDED_CURVE ( )  B_SPLINE_CURVE ( 2, ( #2298, #4315, #1579, #3531, #1670, #4361, #4980, #2387, #7043 ),
 .UNSPECIFIED., .F., .T. ) 
 B_SPLINE_CURVE_WITH_KNOTS ( ( 3, 2, 2, 2, 3 ),
 ( 0.4285714285714284366, 0.4464285714285713413, 0.4642857142857141906, 0.4821428571428570953, 0.4999999999999999445 ),
 .UNSPECIFIED. ) 
 CURVE ( )  GEOMETRIC_REPRESENTATION_ITEM ( )  RATIONAL_B_SPLINE_CURVE ( ( 1.000000000000000444, 0.9238795325112862944, 1.000000000000000000, 0.9238795325112867385, 1.000000000000000000, 0.9238795325112867385, 1.000000000000000000, 0.9238795325112869605, 0.9999999999999997780 ) ) 
 REPRESENTATION_ITEM ( '' )  );
#7334=CARTESIAN_POINT ( 'NONE',  ( -2.796473189345805913E-16, -40.43301269999997061, -95.44999999890752918 ) ) ;
#7342=ORIENTED_EDGE ( 'NONE', *, *, #4705, .F. ) ;
#7346=CARTESIAN_POINT ( 'NONE',  ( 9.184850993605145972E-16, -49.99999999999997158, -100.2999999978150498 ) ) ;
#7347=ADVANCED_FACE ( 'NONE', ( #1756 ), #8493, .T. ) ;
#7348=CARTESIAN_POINT ( 'NONE',  ( -3.061616997868382155E-16, -39.99999999999997158, -95.20000000000000284 ) ) ;
#7349=CARTESIAN_POINT ( 'NONE',  ( -2.071067811865475061, -39.99999999999997158, -98.35000000000000853 ) ) ;
#7352=DIRECTION ( 'NONE',  ( -0.000000000000000000, -0.000000000000000000, -1.000000000000000000 ) ) ;
#7356=CARTESIAN_POINT ( 'NONE',  ( 1.891708078845682595, -40.43301269999998482, -96.49999999890755475 ) ) ;
#7357=CARTESIAN_POINT ( 'NONE',  ( 9.184850993605145972E-16, -49.99999999999997158, -96.29999999781504982 ) ) ;
#7359=CARTESIAN_POINT ( 'NONE',  ( -3.229347689422840784, -41.77065231057713390, -96.94999999890751496 ) ) ;
#7364=CARTESIAN_POINT ( 'NONE',  ( 4.999999999999998224, -44.99999999999997158, -96.19300000002185413 ) ) ;
#7370=CARTESIAN_POINT ( 'NONE',  ( 5.000000000000000000, -47.07106781186545419, -99.45000000000000284 ) ) ;
#7376=CARTESIAN_POINT ( 'NONE',  ( 4.999999999999998224, -44.99999999999997158, -97.00000000000000000 ) ) ;
#7381=CARTESIAN_POINT ( 'NONE',  ( -3.229347689422840784, -41.77065231057713390, -96.14999999890753202 ) ) ;
#7392=CARTESIAN_POINT ( 'NONE',  ( -3.535533905932736864, -41.46446609406723383, -100.5999999978150470 ) ) ;
#7400=CARTESIAN_POINT ( 'NONE',  ( -4.566987299999997418, -46.89170807884566017, -96.99999999890751212 ) ) ;
#7401=CARTESIAN_POINT ( 'NONE',  ( -3.061616997868382155E-16, -39.99999999999997158, -97.49999999781503845 ) ) ;
#7403=CARTESIAN_POINT ( 'NONE',  ( 4.566987299999998307, -43.10829192115428299, -99.59999999890756328 ) ) ;
#7404=APPLICATION_CONTEXT ( 'automotive_design' ) ;
#7407=CARTESIAN_POINT ( 'NONE',  ( -3.535533905932736864, -41.46446609406723383, -95.09300000002185982 ) ) ;
#7410=CARTESIAN_POINT ( 'NONE',  ( 4.999999999999987566, -42.92893218813447476, -96.04999999781503561 ) ) ;
#7413=VERTEX_POINT ( 'NONE', #3293 ) ;
#7418=CARTESIAN_POINT ( 'NONE',  ( -3.535533905932736864, -41.46446609406723383, -96.70000000000000284 ) ) ;
#7430=ORIENTED_EDGE ( 'NONE', *, *, #5462, .F. ) ;
#7436=CARTESIAN_POINT ( 'NONE',  ( -1.891708078845683039, -40.43301269999998482, -95.59999999890753486 ) ) ;
#7438=CARTESIAN_POINT ( 'NONE',  ( -2.071067811865475505, -49.99999999999997158, -96.34999999781506119 ) ) ;
#7443=ORIENTED_EDGE ( 'NONE', *, *, #3113, .T. ) ;
#7444=CARTESIAN_POINT ( 'NONE',  ( -1.891708078845683039, -40.43301269999998482, -96.39999999890753202 ) ) ;
#7445=CARTESIAN_POINT ( 'NONE',  ( 9.184850993605145972E-16, -49.99999999999997158, -99.59999999999999432 ) ) ;
#7447=CARTESIAN_POINT ( 'NONE',  ( -4.566987299999997418, -46.89170807884566727, -97.59999999890756328 ) ) ;
#7449=DIRECTION ( 'NONE',  ( -0.000000000000000000, -0.000000000000000000, -1.000000000000000000 ) ) ;
#7452=CARTESIAN_POINT ( 'NONE',  ( -4.999999999999998224, -44.99999999999997158, -97.39300000002185698 ) ) ;
#7455=DIRECTION ( 'NONE',  ( 0.000000000000000000, -0.000000000000000000, -1.000000000000000000 ) ) ;
#7462=CARTESIAN_POINT ( 'NONE',  ( -4.999999999999998224, -44.99999999999997158, -95.00000000000000000 ) ) ;
#7467=ORIENTED_EDGE ( 'NONE', *, *, #7961, .T. ) ;
#7474=CARTESIAN_POINT ( 'NONE',  ( -3.229347689422839451, -48.22934768942280925, -97.54999999890752349 ) ) ;
#7477=CARTESIAN_POINT ( 'NONE',  ( 2.071067811865474173, -39.99999999999997158, -99.14999999781504414 ) ) ;
#7480=VERTEX_POINT ( 'NONE', #1917 ) ;
#7486=CARTESIAN_POINT ( 'NONE',  ( 4.566987300000000083, -46.89170807884564596, -96.69999999890751496 ) ) ;
#7487=CARTESIAN_POINT ( 'NONE',  ( -2.071067811865475061, -39.99999999999997158, -96.64999999781504414 ) ) ;
#7489=CARTESIAN_POINT ( 'NONE',  ( -3.229347689422839451, -48.22934768942280925, -99.94999999890752918 ) ) ;
#7495=CARTESIAN_POINT ( 'NONE',  ( 4.999999999999998224, -44.99999999999997158, -95.40000000000000568 ) ) ;
#7497=CARTESIAN_POINT ( 'NONE',  ( -3.535533905932736864, -41.46446609406723383, -95.79999999781504982 ) ) ;
#7499=ORIENTED_EDGE ( 'NONE', *, *, #4668, .F. ) ;
#7500=CARTESIAN_POINT ( 'NONE',  ( -4.999999999999997335, -47.07106781186546129, -100.4499999978150413 ) ) ;
#7517=CARTESIAN_POINT ( 'NONE',  ( -3.229347689422840784, -41.77065231057713390, -100.1499999989075320 ) ) ;
#7520=CARTESIAN_POINT ( 'NONE',  ( -4.566987299999998307, -44.99999999999997158, -97.04999999890752349 ) ) ;
#7522=CARTESIAN_POINT ( 'NONE',  ( 5.000000000000009770, -47.07106781186543998, -96.14999999781502993 ) ) ;
#7530=CARTESIAN_POINT ( 'NONE',  ( 3.535533905932736420, -41.46446609406723383, -98.39999999781504414 ) ) ;
#7532=CARTESIAN_POINT ( 'NONE',  ( 1.891708078845685481, -49.56698729999997255, -98.19999999890751496 ) ) ;
#7535=CARTESIAN_POINT ( 'NONE',  ( -3.535533905932735532, -48.53553390593270933, -95.70000000000000284 ) ) ;
#7540=CARTESIAN_POINT ( 'NONE',  ( 3.535533969928884801, -41.46446615806338087, -100.0000000000000142 ) ) ;
#7543=LINE ( 'NONE', #7462, #2054 ) ;
#7547=DIRECTION ( 'NONE',  ( 0.8660254037844382635, 0.000000000000000000, 0.5000000000000005551 ) ) ;
#7550=ORIENTED_EDGE ( 'NONE', *, *, #6788, .F. ) ;
#7552=ORIENTED_EDGE ( 'NONE', *, *, #3963, .F. ) ;
#7558=CARTESIAN_POINT ( 'NONE',  ( -4.566987299999998307, -44.99999999999997158, -96.04999999890752349 ) ) ;
#7561=CARTESIAN_POINT ( 'NONE',  ( -1.891708078845683039, -40.43301269999998482, -98.79999999890753770 ) ) ;
#7573=CARTESIAN_POINT ( 'NONE',  ( -2.071067811865475061, -39.99999999999997158, -99.04999999781504982 ) ) ;
#7574=CARTESIAN_POINT ( 'NONE',  ( 3.535533905932737309, -48.53553390593270933, -97.79999999781504982 ) ) ;
#7575=CARTESIAN_POINT ( 'NONE',  ( 1.891708078845682595, -40.43301269999998482, -99.49999999890754054 ) ) ;
#7579=CARTESIAN_POINT ( 'NONE',  ( 5.000000000000000000, -47.07106781186545419, -98.64300000002185698 ) ) ;
#7581=CARTESIAN_POINT ( 'NONE',  ( -4.566987299999997418, -46.89170807884566727, -96.79999999890753770 ) ) ;
#7599=AXIS2_PLACEMENT_3D ( 'NONE', #7783, #1163, #1753 ) ;
#7600=CARTESIAN_POINT ( 'NONE',  ( -2.796473189345805913E-16, -40.43301269999997061, -97.04999999890752349 ) ) ;
#7604=CARTESIAN_POINT ( 'NONE',  ( -1.891708078845683483, -49.56698729999997255, -96.89999999890751781 ) ) ;
#7608=( BOUNDED_CURVE ( )  B_SPLINE_CURVE ( 2, ( #3957, #8014, #1971, #4659, #7348, #2686, #5353, #6285, #246 ),
 .UNSPECIFIED., .F., .T. ) 
 B_SPLINE_CURVE_WITH_KNOTS ( ( 3, 2, 2, 2, 3 ),
 ( 0.000000000000000000, 0.01785714285714286309, 0.03571428571428572618, 0.05357142857142858927, 0.07142857142857145236 ),
 .UNSPECIFIED. ) 
 CURVE ( )  GEOMETRIC_REPRESENTATION_ITEM ( )  RATIONAL_B_SPLINE_CURVE ( ( 1.000000000000000000, 0.9238795325112867385, 1.000000000000000000, 0.9238795325112867385, 1.000000000000000000, 0.9238795325112867385, 1.000000000000000000, 0.9238795325112866275, 1.000000000000000222 ) ) 
 REPRESENTATION_ITEM ( '' )  );
#7615=CARTESIAN_POINT ( 'NONE',  ( -2.071067811865475505, -49.99999999999996447, -99.54999999781506403 ) ) ;
#7616=CARTESIAN_POINT ( 'NONE',  ( -4.999999999999986677, -47.07106781186546129, -98.04999999781503561 ) ) ;
#7617=CARTESIAN_POINT ( 'NONE',  ( 1.891708078845685481, -49.56698729999997255, -99.79999999890752349 ) ) ;
#7622=CARTESIAN_POINT ( 'NONE',  ( -3.061616997868382155E-16, -39.99999999999997158, -99.19300000002183992 ) ) ;
#7624=CARTESIAN_POINT ( 'NONE',  ( -4.999999999999998224, -42.92893218813448897, -96.54999999781504982 ) ) ;
#7634=CARTESIAN_POINT ( 'NONE',  ( -3.535533905932735532, -48.53553390593270933, -98.10000000000000853 ) ) ;
#7646=CARTESIAN_POINT ( 'NONE',  ( -4.566987299999997418, -46.89170807884566017, -97.59999999890754907 ) ) ;
#7648=CARTESIAN_POINT ( 'NONE',  ( 4.999999999999998224, -44.99999999999997158, -96.89999999781505835 ) ) ;
#7650=CARTESIAN_POINT ( 'NONE',  ( 1.891708078845685481, -49.56698729999997255, -99.19999999890751496 ) ) ;
#7651=CARTESIAN_POINT ( 'NONE',  ( 7.499999999999999112, -44.99999999999997158, -105.0000000000000142 ) ) ;
#7652=CARTESIAN_POINT ( 'NONE',  ( -1.891708078845683483, -49.56698729999997255, -98.49999999890752633 ) ) ;
#7653=CYLINDRICAL_SURFACE ( 'NONE', #2695, 4.999999999999998224 ) ;
#7654=VERTEX_POINT ( 'NONE', #4605 ) ;
#7660=CARTESIAN_POINT ( 'NONE',  ( -4.999999999999998224, -44.99999999999997158, -99.69999999781505551 ) ) ;
#7661=CARTESIAN_POINT ( 'NONE',  ( -3.229347689422840784, -41.77065231057713390, -99.54999999890752349 ) ) ;
#7663=CARTESIAN_POINT ( 'NONE',  ( 2.071067811865474173, -39.99999999999997158, -99.14999999781504414 ) ) ;
#7665=CARTESIAN_POINT ( 'NONE',  ( -3.229347689422839451, -48.22934768942280925, -97.54999999890752349 ) ) ;
#7668=CARTESIAN_POINT ( 'NONE',  ( -4.999999999999998224, -46.91341716182541433, -94.95380602337444031 ) ) ;
#7670=CARTESIAN_POINT ( 'NONE',  ( 1.891708078845685481, -49.56698729999997255, -95.79999999890752349 ) ) ;
#7671=CARTESIAN_POINT ( 'NONE',  ( 2.071067811865474173, -39.99999999999997158, -95.94999999781504130 ) ) ;
#7674=CARTESIAN_POINT ( 'NONE',  ( -4.999999999999998224, -44.99999999999997158, -100.4999999978150385 ) ) ;
#7678=CARTESIAN_POINT ( 'NONE',  ( -1.891708078845683705, -49.56698729999997255, -96.09999999890752065 ) ) ;
#7679=CARTESIAN_POINT ( 'NONE',  ( -3.061616997868382155E-16, -39.99999999999997158, -98.40000000000000568 ) ) ;
#7688=ORIENTED_EDGE ( 'NONE', *, *, #515, .F. ) ;
#7695=CARTESIAN_POINT ( 'NONE',  ( -1.891708078845683039, -40.43301269999998482, -98.59999999890754907 ) ) ;
#7699=CARTESIAN_POINT ( 'NONE',  ( 1.891708078845682595, -40.43301269999998482, -96.49999999890752633 ) ) ;
#7700=CARTESIAN_POINT ( 'NONE',  ( 4.566987300000000083, -46.89170807884565306, -96.69999999890752918 ) ) ;
#7701=EDGE_CURVE ( 'NONE', #6319, #71, #6696, .T. ) ;
#7712=CARTESIAN_POINT ( 'NONE',  ( -4.999999999999998224, -44.99999999999997158, -97.29999999781504982 ) ) ;
#7714=AXIS2_PLACEMENT_3D ( 'NONE', #434, #6402, #5828 ) ;
#7715=CARTESIAN_POINT ( 'NONE',  ( 3.535533905932737309, -48.53553390593270933, -97.90000000000000568 ) ) ;
#7721=CARTESIAN_POINT ( 'NONE',  ( -3.535533905932735532, -48.53553390593270933, -97.19999999781504130 ) ) ;
#7727=CARTESIAN_POINT ( 'NONE',  ( 1.891708078845685481, -49.56698729999997255, -95.99999999890751212 ) ) ;
#7733=ORIENTED_EDGE ( 'NONE', *, *, #3105, .F. ) ;
#7737=CARTESIAN_POINT ( 'NONE',  ( 8.389419568037416259E-16, -49.56698729999997255, -98.24999999890752633 ) ) ;
#7738=UNCERTAINTY_MEASURE_WITH_UNIT (LENGTH_MEASURE( 1.000000000000000082E-05 ), #896, 'distance_accuracy_value', 'NONE');
#7743=CARTESIAN_POINT ( 'NONE',  ( 3.229347689422841228, -48.22934768942280925, -95.94999999890751496 ) ) ;
#7748=ORIENTED_EDGE ( 'NONE', *, *, #7287, .T. ) ;
#7751=CYLINDRICAL_SURFACE ( 'NONE', #7852, 4.999999999999998224 ) ;
#7753=CARTESIAN_POINT ( 'NONE',  ( -2.071067811865475505, -49.99999999999997158, -95.65000000000000568 ) ) ;
#7755=CARTESIAN_POINT ( 'NONE',  ( 2.071067811865477282, -49.99999999999996447, -97.95000000000000284 ) ) ;
#7761=CARTESIAN_POINT ( 'NONE',  ( -4.999999999999998224, -42.92893218813448897, -98.25000000000000000 ) ) ;
#7762=CARTESIAN_POINT ( 'NONE',  ( 4.999999999999998224, -44.99999999999997158, -96.89999999781505835 ) ) ;
#7774=ORIENTED_EDGE ( 'NONE', *, *, #786, .T. ) ;
#7779=CARTESIAN_POINT ( 'NONE',  ( -1.891708078845683039, -40.43301269999998482, -99.39999999890751781 ) ) ;
#7783=CARTESIAN_POINT ( 'NONE',  ( 0.000000000000000000, -44.99999999999997158, -105.0000000000000142 ) ) ;
#7786=CARTESIAN_POINT ( 'NONE',  ( -3.229347689422840784, -41.77065231057713390, -97.14999999890753202 ) ) ;
#7787=CARTESIAN_POINT ( 'NONE',  ( 0.000000000000000000, 0.000000000000000000, 0.000000000000000000 ) ) ;
#7796=DIRECTION ( 'NONE',  ( -0.000000000000000000, -0.000000000000000000, -1.000000000000000000 ) ) ;
#7798=DIRECTION ( 'NONE',  ( -0.000000000000000000, -0.000000000000000000, -1.000000000000000000 ) ) ;
#7800=CARTESIAN_POINT ( 'NONE',  ( 4.999999999999998224, -44.99999999999997158, -96.20000000000000284 ) ) ;
#7806=ORIENTED_EDGE ( 'NONE', *, *, #2361, .F. ) ;
#7807=CARTESIAN_POINT ( 'NONE',  ( -4.999999999999998224, -44.99999999999997158, -99.00000000000000000 ) ) ;
#7809=CARTESIAN_POINT ( 'NONE',  ( 3.535533905932737309, -48.53553390593270933, -96.99999999781503845 ) ) ;
#7810=CARTESIAN_POINT ( 'NONE',  ( -3.570038910208443106, -48.51199280350586207, -100.0000267679173760 ) ) ;
#7812=FACE_OUTER_BOUND ( 'NONE', #634, .T. ) ;
#7816=CYLINDRICAL_SURFACE ( 'NONE', #7990, 4.999999999999998224 ) ;
#7824=CARTESIAN_POINT ( 'NONE',  ( 3.229347689422839895, -41.77065231057713390, -99.54999999890752349 ) ) ;
#7827=CARTESIAN_POINT ( 'NONE',  ( 1.891708078845682595, -40.43301269999998482, -99.69999999890752918 ) ) ;
#7829=CARTESIAN_POINT ( 'NONE',  ( -4.566987299999997418, -46.89170807884566727, -96.99999999890751212 ) ) ;
#7832=VERTEX_POINT ( 'NONE', #5997 ) ;
#7835=ORIENTED_EDGE ( 'NONE', *, *, #793, .F. ) ;
#7839=CARTESIAN_POINT ( 'NONE',  ( 3.535533905932737309, -48.53553390593270933, -95.50000000000000000 ) ) ;
#7841=CARTESIAN_POINT ( 'NONE',  ( -4.999999999999998224, -42.92893218813448897, -95.04999999999999716 ) ) ;
#7847=CARTESIAN_POINT ( 'NONE',  ( -3.535533905932735532, -48.53553390593270933, -97.29999999999999716 ) ) ;
#7851=DIRECTION ( 'NONE',  ( -0.000000000000000000, -0.000000000000000000, -1.000000000000000000 ) ) ;
#7852=AXIS2_PLACEMENT_3D ( 'NONE', #1048, #7796, #339 ) ;
#7865=CARTESIAN_POINT ( 'NONE',  ( -3.535533905932736864, -41.46446609406723383, -95.90000000000000568 ) ) ;
#7871=CARTESIAN_POINT ( 'NONE',  ( 4.566987299999998307, -44.99999999999997158, -99.84999999890752065 ) ) ;
#7874=LINE ( 'NONE', #7165, #4550 ) ;
#7878=VERTEX_POINT ( 'NONE', #8563 ) ;
#7883=CARTESIAN_POINT ( 'NONE',  ( 5.000000000000003553, -42.92893218813449607, -97.64999999781502993 ) ) ;
#7885=CARTESIAN_POINT ( 'NONE',  ( 5.000000000000000000, -47.07106781186545419, -97.04999999999999716 ) ) ;
#7890=CARTESIAN_POINT ( 'NONE',  ( 4.999999999999998224, -44.99999999999997158, -98.60000000000000853 ) ) ;
#7913=CARTESIAN_POINT ( 'NONE',  ( -4.566987299999998307, -44.99999999999997158, -99.44999999890752918 ) ) ;
#7924=CARTESIAN_POINT ( 'NONE',  ( -2.071067811865475061, -39.99999999999997158, -99.14999999999999147 ) ) ;
#7927=EDGE_LOOP ( 'NONE', ( #7467, #7774, #6863, #3991 ) ) ;
#7931=CARTESIAN_POINT ( 'NONE',  ( -3.535533905932735532, -48.53553390593270933, -96.50000000000000000 ) ) ;
#7933=CARTESIAN_POINT ( 'NONE',  ( -4.566987299999998307, -43.10829192115428299, -97.69999999890751496 ) ) ;
#7934=CARTESIAN_POINT ( 'NONE',  ( 4.966556519403932946, -45.64283254358549158, -99.99918711676903627 ) ) ;
#7938=CARTESIAN_POINT ( 'NONE',  ( 3.535533905932737309, -48.53553390593270933, -96.99999999781503845 ) ) ;
#7939=( BOUNDED_CURVE ( )  B_SPLINE_CURVE ( 2, ( #5722, #7130, #7839, #8424, #3788, #7753, #4404, #4487, #1093 ),
 .UNSPECIFIED., .F., .T. ) 
 B_SPLINE_CURVE_WITH_KNOTS ( ( 3, 2, 2, 2, 3 ),
 ( 0.07142857142857145236, 0.08928571428571430157, 0.1071428571428571369, 0.1249999999999999861, 0.1428571428571428215 ),
 .UNSPECIFIED. ) 
 CURVE ( )  GEOMETRIC_REPRESENTATION_ITEM ( )  RATIONAL_B_SPLINE_CURVE ( ( 0.9999999999999998890, 0.9238795325112868495, 1.000000000000000000, 0.9238795325112867385, 1.000000000000000000, 0.9238795325112867385, 1.000000000000000000, 0.9238795325112868495, 0.9999999999999998890 ) ) 
 REPRESENTATION_ITEM ( '' )  );
#7942=CARTESIAN_POINT ( 'NONE',  ( 4.999999999999998224, -44.99999999999997158, -97.79999999999999716 ) ) ;
#7955=CARTESIAN_POINT ( 'NONE',  ( -4.566987299999997418, -46.89170807884566727, -98.59999999890753486 ) ) ;
#7961=EDGE_CURVE ( 'NONE', #196, #5319, #5910, .T. ) ;
#7962=ORIENTED_EDGE ( 'NONE', *, *, #2371, .T. ) ;
#7965=ADVANCED_FACE ( 'NONE', ( #797 ), #2132, .F. ) ;
#7968=CARTESIAN_POINT ( 'NONE',  ( -3.535533905932736864, -41.46446609406723383, -99.79999999781504982 ) ) ;
#7970=CARTESIAN_POINT ( 'NONE',  ( 4.999999999999998224, -42.92893218813448897, -99.35000000000000853 ) ) ;
#7977=CARTESIAN_POINT ( 'NONE',  ( -4.783493649999997821, -44.99999999999997158, -95.12499999945376317 ) ) ;
#7978=CARTESIAN_POINT ( 'NONE',  ( 4.999999999999998224, -44.99999999999997158, -96.89999999781505835 ) ) ;
#7980=CARTESIAN_POINT ( 'NONE',  ( -1.891708078845683039, -40.43301269999998482, -98.59999999890754907 ) ) ;
#7982=CARTESIAN_POINT ( 'NONE',  ( 5.004075312705366763, -44.80061875307438157, -100.0004355954672093 ) ) ;
#7986=CARTESIAN_POINT ( 'NONE',  ( -3.535533905932736864, -41.46446609406723383, -97.49300000002185129 ) ) ;
#7990=AXIS2_PLACEMENT_3D ( 'NONE', #6526, #3066, #6481 ) ;
#7996=( BOUNDED_CURVE ( )  B_SPLINE_CURVE ( 2, ( #7540, #269, #800, #5556, #5646, #8262, #1502, #2312, #4197, #7500, #7674, #1639, #2224, #4331, #7011 ),
 .UNSPECIFIED., .F., .T. ) 
 B_SPLINE_CURVE_WITH_KNOTS ( ( 3, 2, 2, 2, 2, 2, 2, 3 ),
 ( 0.7678571432794624174, 0.7857142857142856984, 0.8035714285714286031, 0.8214285714285713969, 0.8392857142857143016, 0.8571428571428570953, 0.8750000000000000000, 0.8928571428571429047 ),
 .UNSPECIFIED. ) 
 CURVE ( )  GEOMETRIC_REPRESENTATION_ITEM ( )  RATIONAL_B_SPLINE_CURVE ( ( 1.000000000000000000, 0.9238795325112867385, 1.000000000000000000, 0.9238795325112867385, 1.000000000000000000, 0.9238795325112867385, 1.000000000000000000, 0.9238795325112867385, 1.000000000000000000, 0.9238795325112867385, 1.000000000000000000, 0.9238795325112867385, 1.000000000000000000, 0.9238795325112867385, 1.000000000000000000 ) ) 
 REPRESENTATION_ITEM ( '' )  );
#8002=CARTESIAN_POINT ( 'NONE',  ( -4.566987299999997418, -46.89170807884566727, -100.1999999989075150 ) ) ;
#8004=CARTESIAN_POINT ( 'NONE',  ( -4.999999999999998224, -44.99999999999997158, -99.00000000000000000 ) ) ;
#8010=ORIENTED_EDGE ( 'NONE', *, *, #723, .F. ) ;
#8013=CARTESIAN_POINT ( 'NONE',  ( -2.071067811865475061, -39.99999999999997158, -98.24999999781506688 ) ) ;
#8014=CARTESIAN_POINT ( 'NONE',  ( -4.999999999999998224, -42.92893218813449607, -95.04999999999999716 ) ) ;
#8015=CARTESIAN_POINT ( 'NONE',  ( -3.535533905932735532, -48.53553390593270933, -98.90000000000000568 ) ) ;
#8020=CARTESIAN_POINT ( 'NONE',  ( 3.229347689422841228, -48.22934768942280925, -97.54999999890752349 ) ) ;
#8021=CARTESIAN_POINT ( 'NONE',  ( 3.535533905932736420, -41.46446609406723383, -95.99999999781503845 ) ) ;
#8023=CARTESIAN_POINT ( 'NONE',  ( 3.229347689422841228, -48.22934768942280925, -98.14999999890753202 ) ) ;
#8027=CARTESIAN_POINT ( 'NONE',  ( -3.061616997868382155E-16, -39.99999999999997158, -96.79300000002184845 ) ) ;
#8029=VECTOR ( 'NONE', #7547, 1000.000000000000114 ) ;
#8031=CARTESIAN_POINT ( 'NONE',  ( -3.535533905932736864, -41.46446609406723383, -97.50000000000000000 ) ) ;
#8034=ORIENTED_EDGE ( 'NONE', *, *, #5114, .T. ) ;
#8043=CARTESIAN_POINT ( 'NONE',  ( -3.229347689422839451, -48.22934768942280925, -95.94999999890752918 ) ) ;
#8045=ORIENTED_EDGE ( 'NONE', *, *, #6388, .F. ) ;
#8055=CARTESIAN_POINT ( 'NONE',  ( -4.999999999999998224, -42.92893218813448897, -99.74999999781503845 ) ) ;
#8064=CARTESIAN_POINT ( 'NONE',  ( 8.389419568037416259E-16, -49.56698729999997255, -97.64999999890751781 ) ) ;
#8066=CARTESIAN_POINT ( 'NONE',  ( 9.184850993605145972E-16, -49.99999999999997158, -97.09999999781504698 ) ) ;
#8068=CARTESIAN_POINT ( 'NONE',  ( 1.891708078845685481, -49.56698729999997255, -98.19999999890751496 ) ) ;
#8075=CARTESIAN_POINT ( 'NONE',  ( 2.071067811865477282, -49.99999999999996447, -97.14300000002185698 ) ) ;
#8078=CARTESIAN_POINT ( 'NONE',  ( 3.535533905932736420, -41.46446609406723383, -97.69999999999998863 ) ) ;
#8093=CARTESIAN_POINT ( 'NONE',  ( -3.229347689422839451, -48.22934768942280925, -96.74999999890752633 ) ) ;
#8102=ORIENTED_EDGE ( 'NONE', *, *, #2327, .T. ) ;
#8106=CARTESIAN_POINT ( 'NONE',  ( -3.535533905932735532, -48.53553390593270933, -99.59999999781504698 ) ) ;
#8115=CARTESIAN_POINT ( 'NONE',  ( 1.891708078845682595, -40.43301269999998482, -98.09999999890752065 ) ) ;
#8116=CARTESIAN_POINT ( 'NONE',  ( 3.535533905932736420, -41.46446609406723383, -96.79999999781504982 ) ) ;
#8118=CARTESIAN_POINT ( 'NONE',  ( 3.229347689422841228, -48.22934768942280925, -98.94999999890752918 ) ) ;
#8119=DIRECTION ( 'NONE',  ( -1.000000000000000000, 0.000000000000000000, 0.000000000000000000 ) ) ;
#8123=CARTESIAN_POINT ( 'NONE',  ( -3.535533905932736864, -41.46446609406723383, -95.89300000002184277 ) ) ;
#8128=ORIENTED_EDGE ( 'NONE', *, *, #7144, .F. ) ;
#8130=VECTOR ( 'NONE', #1284, 1000.000000000000000 ) ;
#8139=DIRECTION ( 'NONE',  ( 1.000000000000000000, 0.000000000000000000, -0.000000000000000000 ) ) ;
#8140=CARTESIAN_POINT ( 'NONE',  ( -3.535533905932735532, -48.53553390593270933, -99.59999999781504698 ) ) ;
#8151=CARTESIAN_POINT ( 'NONE',  ( -7.654042494670954648E-16, -39.99999999999997158, -100.0000000000000000 ) ) ;
#8153=CARTESIAN_POINT ( 'NONE',  ( 1.891708078845685481, -49.56698729999997255, -95.99999999890751212 ) ) ;
#8161=CARTESIAN_POINT ( 'NONE',  ( 1.891708078845685481, -49.56698729999997255, -98.39999999890753202 ) ) ;
#8162=CARTESIAN_POINT ( 'NONE',  ( 5.000000000000000000, -47.07106781186545419, -96.14999999781504414 ) ) ;
#8163=CARTESIAN_POINT ( 'NONE',  ( 2.071067811865477282, -49.99999999999997158, -97.84999999781504698 ) ) ;
#8164=CARTESIAN_POINT ( 'NONE',  ( 3.229347689422841228, -48.22934768942280925, -99.74999999890752633 ) ) ;
#8167=CARTESIAN_POINT ( 'NONE',  ( 4.999999999999998224, -42.92893218813448897, -95.34999999999999432 ) ) ;
#8181=LINE ( 'NONE', #4872, #8029 ) ;
#8183=SURFACE_SIDE_STYLE ('',( #4782 ) ) ;
#8184=ORIENTED_EDGE ( 'NONE', *, *, #6788, .T. ) ;
#8191=EDGE_LOOP ( 'NONE', ( #4141, #6163, #398, #4565 ) ) ;
#8193=CARTESIAN_POINT ( 'NONE',  ( 4.566987299999998307, -43.10829192115428299, -96.39999999890753202 ) ) ;
#8195=DIRECTION ( 'NONE',  ( -1.000000000000000000, 0.000000000000000000, 0.000000000000000000 ) ) ;
#8196=CARTESIAN_POINT ( 'NONE',  ( -1.891708078845683483, -49.56698729999997255, -96.09999999890750644 ) ) ;
#8207=CARTESIAN_POINT ( 'NONE',  ( 4.566987299999998307, -44.99999999999997158, -98.24999999890751212 ) ) ;
#8208=CARTESIAN_POINT ( 'NONE',  ( 1.932551333443697450, -39.99999999999997158, -100.7466559142068832 ) ) ;
#8210=CARTESIAN_POINT ( 'NONE',  ( -4.566987299999997418, -46.89170807884566727, -99.19999999890751496 ) ) ;
#8214=CARTESIAN_POINT ( 'NONE',  ( 2.071067811865477282, -49.99999999999996447, -95.54999999999999716 ) ) ;
#8216=CARTESIAN_POINT ( 'NONE',  ( -3.229347689422839451, -48.22934768942280925, -95.94999999890752918 ) ) ;
#8235=VECTOR ( 'NONE', #3166, 1000.000000000000000 ) ;
#8237=CARTESIAN_POINT ( 'NONE',  ( 4.566987300000000083, -46.89170807884564596, -96.49999999890755475 ) ) ;
#8238=CARTESIAN_POINT ( 'NONE',  ( -4.999999999999987566, -42.92893218813447476, -99.84999999999999432 ) ) ;
#8240=CARTESIAN_POINT ( 'NONE',  ( -4.566987299999998307, -44.99999999999997158, -98.64999999890751781 ) ) ;
#8242=CYLINDRICAL_SURFACE ( 'NONE', #4596, 4.999999999999998224 ) ;
#8243=( BOUNDED_CURVE ( )  B_SPLINE_CURVE ( 2, ( #2571, #5329, #8031, #5244, #6039, #3365, #8078, #2524, #7942 ),
 .UNSPECIFIED., .F., .T. ) 
 B_SPLINE_CURVE_WITH_KNOTS ( ( 3, 2, 2, 2, 3 ),
 ( 0.4285714285714286031, 0.4464285714285715079, 0.4642857142857143016, 0.4821428571428571508, 0.5000000000000000000 ),
 .UNSPECIFIED. ) 
 CURVE ( )  GEOMETRIC_REPRESENTATION_ITEM ( )  RATIONAL_B_SPLINE_CURVE ( ( 0.9999999999999997780, 0.9238795325112869605, 1.000000000000000000, 0.9238795325112867385, 1.000000000000000000, 0.9238795325112867385, 1.000000000000000000, 0.9238795325112867385, 1.000000000000000000 ) ) 
 REPRESENTATION_ITEM ( '' )  );
#8249=CARTESIAN_POINT ( 'NONE',  ( 5.000000000000004441, -47.07106781186543998, -98.54999999781504982 ) ) ;
#8250=CARTESIAN_POINT ( 'NONE',  ( 8.389419568037416259E-16, -49.56698729999997255, -100.0499999989075093 ) ) ;
#8251=CARTESIAN_POINT ( 'NONE',  ( -4.999999999999997335, -47.07106781186546129, -100.4499999978150413 ) ) ;
#8253=CARTESIAN_POINT ( 'NONE',  ( 1.891708078845682595, -40.43301269999998482, -98.69999999890752918 ) ) ;
#8256=VECTOR ( 'NONE', #5905, 1000.000000000000000 ) ;
#8257=CARTESIAN_POINT ( 'NONE',  ( -4.999999999999998224, -44.99999999999997158, -99.79300000002184845 ) ) ;
#8258=CARTESIAN_POINT ( 'NONE',  ( 8.389419568037416259E-16, -49.56698729999997255, -96.64999999890753202 ) ) ;
#8260=CARTESIAN_POINT ( 'NONE',  ( -4.783493649999997821, -44.99999999999997158, -95.12499999945376317 ) ) ;
#8262=CARTESIAN_POINT ( 'NONE',  ( 2.071067811865477282, -49.99999999999997158, -100.2499999978150527 ) ) ;
#8269=CARTESIAN_POINT ( 'NONE',  ( -2.071067811865475505, -49.99999999999997158, -99.54999999781504982 ) ) ;
#8278=EDGE_LOOP ( 'NONE', ( #1771, #7099, #6895, #7499 ) ) ;
#8279=CARTESIAN_POINT ( 'NONE',  ( -4.566987299999998307, -43.10829192115428299, -100.0999999989075349 ) ) ;
#8283=CARTESIAN_POINT ( 'NONE',  ( 3.229347689422841228, -48.22934768942280925, -99.14999999890751781 ) ) ;
#8293=CARTESIAN_POINT ( 'NONE',  ( 1.891708078845685481, -49.56698729999997255, -99.99999999890751212 ) ) ;
#8294=CARTESIAN_POINT ( 'NONE',  ( -3.535533905932735532, -48.53553390593270933, -97.99999999781503845 ) ) ;
#8296=CARTESIAN_POINT ( 'NONE',  ( -1.891708078845683039, -40.43301269999998482, -99.39999999890751781 ) ) ;
#8299=CARTESIAN_POINT ( 'NONE',  ( -2.071067811865475061, -39.99999999999997158, -98.34300000002185982 ) ) ;
#8300=CARTESIAN_POINT ( 'NONE',  ( 3.229347689422839895, -41.77065231057713390, -95.54999999890752349 ) ) ;
#8301=CARTESIAN_POINT ( 'NONE',  ( -2.071067811865475505, -49.99999999999996447, -97.14999999781504414 ) ) ;
#8307=CARTESIAN_POINT ( 'NONE',  ( 0.000000000000000000, -44.99999999999997158, -95.00000000000000000 ) ) ;
#8313=EDGE_LOOP ( 'NONE', ( #8481, #3784, #6977, #4136 ) ) ;
#8320=CARTESIAN_POINT ( 'NONE',  ( -4.566987299999997418, -46.89170807884566017, -96.79999999890752349 ) ) ;
#8321=CARTESIAN_POINT ( 'NONE',  ( -7.654042494670954648E-16, -39.99999999999997158, -100.0000000000000000 ) ) ;
#8323=CARTESIAN_POINT ( 'NONE',  ( 1.891708078845682595, -40.43301269999998482, -98.89999999890751781 ) ) ;
#8329=ORIENTED_EDGE ( 'NONE', *, *, #4797, .F. ) ;
#8332=CARTESIAN_POINT ( 'NONE',  ( -4.566987299999998307, -43.10829192115428299, -100.2999999989075093 ) ) ;
#8333=CARTESIAN_POINT ( 'NONE',  ( -3.535533905932736864, -41.46446609406723383, -98.19999999781505551 ) ) ;
#8336=CARTESIAN_POINT ( 'NONE',  ( 3.229347689422839895, -41.77065231057713390, -97.14999999890753202 ) ) ;
#8341=CARTESIAN_POINT ( 'NONE',  ( -4.999999999999998224, -42.92893218813448897, -99.84300000002184561 ) ) ;
#8343=CARTESIAN_POINT ( 'NONE',  ( 2.071067811865477282, -49.99999999999996447, -96.24999999781505267 ) ) ;
#8351=DIRECTION ( 'NONE',  ( 1.000000000000000000, 0.000000000000000000, 0.000000000000000000 ) ) ;
#8364=CARTESIAN_POINT ( 'NONE',  ( 3.229347689422839895, -41.77065231057713390, -97.14999999890753202 ) ) ;
#8365=VECTOR ( 'NONE', #8622, 1000.000000000000000 ) ;
#8369=CARTESIAN_POINT ( 'NONE',  ( 4.566987300000000083, -46.89170807884565306, -97.49999999890754054 ) ) ;
#8371=CARTESIAN_POINT ( 'NONE',  ( 1.891708078845685481, -49.56698729999997255, -96.79999999890753770 ) ) ;
#8381=CARTESIAN_POINT ( 'NONE',  ( -3.061616997868382155E-16, -39.99999999999997158, -100.0624999997268958 ) ) ;
#8382=CARTESIAN_POINT ( 'NONE',  ( -4.999999999999998224, -42.92893218813448897, -99.74999999781503845 ) ) ;
#8384=CARTESIAN_POINT ( 'NONE',  ( -4.999999999999998224, -42.92893218813448897, -96.64999999999999147 ) ) ;
#8388=UNCERTAINTY_MEASURE_WITH_UNIT (LENGTH_MEASURE( 1.000000000000000082E-05 ), #4077, 'distance_accuracy_value', 'NONE');
#8389=CARTESIAN_POINT ( 'NONE',  ( -4.566987299999998307, -44.99999999999997158, -96.04999999890752349 ) ) ;
#8390=CARTESIAN_POINT ( 'NONE',  ( -2.071067811865475061, -39.99999999999997158, -95.84999999781503277 ) ) ;
#8395=VECTOR ( 'NONE', #2558, 1000.000000000000114 ) ;
#8396=CARTESIAN_POINT ( 'NONE',  ( -2.796473189345805913E-16, -40.43301269999997061, -95.64999999890753202 ) ) ;
#8397=CARTESIAN_POINT ( 'NONE',  ( 0.000000000000000000, -44.99999999999997158, -105.0000000000000142 ) ) ;
#8408=CARTESIAN_POINT ( 'NONE',  ( 4.566987300000000083, -46.89170807884564596, -98.89999999890753202 ) ) ;
#8411=VECTOR ( 'NONE', #6409, 1000.000000000000000 ) ;
#8412=CARTESIAN_POINT ( 'NONE',  ( 1.891708078845685481, -49.56698729999997255, -99.99999999890751212 ) ) ;
#8414=CARTESIAN_POINT ( 'NONE',  ( 1.891708078845685481, -49.56698729999997255, -97.59999999890754907 ) ) ;
#8422=CARTESIAN_POINT ( 'NONE',  ( -3.535533905932736864, -41.46446609406723383, -96.59999999781504698 ) ) ;
#8423=CARTESIAN_POINT ( 'NONE',  ( 4.999999999999998224, -44.99999999999997158, -95.00000000000000000 ) ) ;
#8424=CARTESIAN_POINT ( 'NONE',  ( 2.071067811865477282, -49.99999999999997158, -95.54999999999999716 ) ) ;
#8426=CARTESIAN_POINT ( 'NONE',  ( -2.071067811865475061, -39.99999999999997158, -97.54999999999998295 ) ) ;
#8430=CARTESIAN_POINT ( 'NONE',  ( 3.535533905932737309, -48.53553390593270933, -98.70000000000000284 ) ) ;
#8436=CARTESIAN_POINT ( 'NONE',  ( -4.999999999999998224, -42.92893218813449607, -99.74999999781503845 ) ) ;
#8444=EDGE_LOOP ( 'NONE', ( #8586, #3442, #681, #7733 ) ) ;
#8452=CYLINDRICAL_SURFACE ( 'NONE', #7599, 7.499999999999999112 ) ;
#8456=CARTESIAN_POINT ( 'NONE',  ( 4.999999999999998224, -44.99999999999997158, -95.00000000000000000 ) ) ;
#8462=CARTESIAN_POINT ( 'NONE',  ( 0.000000000000000000, -44.99999999999997158, -95.00000000000000000 ) ) ;
#8464=EDGE_CURVE ( 'NONE', #7480, #2692, #3803, .T. ) ;
#8467=CARTESIAN_POINT ( 'NONE',  ( -4.999999999999997335, -47.07106781186546129, -95.75000000000000000 ) ) ;
#8471=CARTESIAN_POINT ( 'NONE',  ( -3.535533905932736864, -41.46446609406723383, -96.70000000000000284 ) ) ;
#8472=CARTESIAN_POINT ( 'NONE',  ( -3.535533905932736864, -41.46446609406723383, -96.59999999781504698 ) ) ;
#8475=CARTESIAN_POINT ( 'NONE',  ( -4.999999999999998224, -44.99999999999997158, -97.40000000000000568 ) ) ;
#8476=CARTESIAN_POINT ( 'NONE',  ( 3.535533969928884801, -41.46446615806338087, -100.0000000000000142 ) ) ;
#8481=ORIENTED_EDGE ( 'NONE', *, *, #2361, .T. ) ;
#8486=CARTESIAN_POINT ( 'NONE',  ( 3.229347689422841228, -48.22934768942280925, -98.14999999890753202 ) ) ;
#8489=CARTESIAN_POINT ( 'NONE',  ( -3.229347689422839451, -48.22934768942280925, -99.34999999890752065 ) ) ;
#8492=CARTESIAN_POINT ( 'NONE',  ( -1.891708078845683039, -40.43301269999998482, -97.99999999890752633 ) ) ;
#8493=CYLINDRICAL_SURFACE ( 'NONE', #2978, 4.999999999999998224 ) ;
#8494=ORIENTED_EDGE ( 'NONE', *, *, #1630, .F. ) ;
#8506=CARTESIAN_POINT ( 'NONE',  ( -3.535533905932736864, -41.46446609406723383, -95.90000000000000568 ) ) ;
#8512=CARTESIAN_POINT ( 'NONE',  ( -3.061616997868382155E-16, -39.99999999999997158, -96.79999999999999716 ) ) ;
#8516=FACE_OUTER_BOUND ( 'NONE', #6026, .T. ) ;
#8525=CARTESIAN_POINT ( 'NONE',  ( -4.566987299999998307, -43.10829192115428299, -98.49999999890752633 ) ) ;
#8529=CARTESIAN_POINT ( 'NONE',  ( -1.891708078845683483, -49.56698729999997255, -99.29999999890752349 ) ) ;
#8531=CARTESIAN_POINT ( 'NONE',  ( 4.566987300000000083, -46.89170807884565306, -97.49999999890754054 ) ) ;
#8543=CARTESIAN_POINT ( 'NONE',  ( -4.999999999999998224, -44.99999999999997158, -98.19999999999998863 ) ) ;
#8546=CARTESIAN_POINT ( 'NONE',  ( 3.535533905932736420, -41.46446609406723383, -97.69999999999998863 ) ) ;
#8547=EDGE_LOOP ( 'NONE', ( #1323, #4466, #305, #6720 ) ) ;
#8553=ADVANCED_FACE ( 'NONE', ( #4765 ), #7653, .T. ) ;
#8554=CARTESIAN_POINT ( 'NONE',  ( -2.071067811865475061, -39.99999999999997158, -98.35000000000000853 ) ) ;
#8555=CARTESIAN_POINT ( 'NONE',  ( 3.215378252671984072, -48.83965459759100725, -99.99931211326003222 ) ) ;
#8562=CARTESIAN_POINT ( 'NONE',  ( -4.999999999999998224, -44.99999999999997158, -96.60000000000000853 ) ) ;
#8563=CARTESIAN_POINT ( 'NONE',  ( 7.499999999999999112, -44.99999999999997158, -100.0000000000000000 ) ) ;
#8568=CARTESIAN_POINT ( 'NONE',  ( -2.071067811865475061, -39.99999999999997158, -96.75000000000001421 ) ) ;
#8574=CARTESIAN_POINT ( 'NONE',  ( -1.891708078845683039, -40.43301269999998482, -99.59999999890754907 ) ) ;
#8579=EDGE_LOOP ( 'NONE', ( #7193, #8329 ) ) ;
#8580=ORIENTED_EDGE ( 'NONE', *, *, #3272, .T. ) ;
#8585=CARTESIAN_POINT ( 'NONE',  ( 2.071067811865477282, -49.99999999999996447, -99.54999999999998295 ) ) ;
#8586=ORIENTED_EDGE ( 'NONE', *, *, #257, .T. ) ;
#8587=APPLICATION_CONTEXT ( 'automotive_design' ) ;
#8593=LINE ( 'NONE', #7977, #8395 ) ;
#8594=CARTESIAN_POINT ( 'NONE',  ( 9.184850993605145972E-16, -49.99999999999997158, -96.40000000000000568 ) ) ;
#8596=CARTESIAN_POINT ( 'NONE',  ( -2.796473189345805913E-16, -40.43301269999997061, -98.64999999890753202 ) ) ;
#8597=CARTESIAN_POINT ( 'NONE',  ( -4.988661577999454089, -45.44142994503554434, -100.0006878868518783 ) ) ;
#8610=EDGE_CURVE ( 'NONE', #6319, #5143, #954, .T. ) ;
#8611=( BOUNDED_CURVE ( )  B_SPLINE_CURVE ( 2, ( #910, #7522, #2288, #3606, #2948, #7438, #6767, #2818, #3480 ),
 .UNSPECIFIED., .F., .T. ) 
 B_SPLINE_CURVE_WITH_KNOTS ( ( 3, 2, 2, 2, 3 ),
 ( 0.07142857142857131358, 0.08928571428571420443, 0.1071428571428570814, 0.1249999999999999722, 0.1428571428571428492 ),
 .UNSPECIFIED. ) 
 CURVE ( )  GEOMETRIC_REPRESENTATION_ITEM ( )  RATIONAL_B_SPLINE_CURVE ( ( 1.000000000000000444, 0.9238795325112862944, 1.000000000000000000, 0.9238795325112867385, 1.000000000000000000, 0.9238795325112867385, 1.000000000000000000, 0.9238795325112867385, 1.000000000000000000 ) ) 
 REPRESENTATION_ITEM ( '' )  );
#8619=CARTESIAN_POINT ( 'NONE',  ( 3.229347689422841228, -48.22934768942280925, -99.14999999890751781 ) ) ;
#8621=EDGE_LOOP ( 'NONE', ( #7342, #6975 ) ) ;
#8622=DIRECTION ( 'NONE',  ( -0.000000000000000000, -0.000000000000000000, -1.000000000000000000 ) ) ;
#8631=CARTESIAN_POINT ( 'NONE',  ( -3.535533905932735532, -48.53553390593270933, -100.3999999978150441 ) ) ;
#8633=CARTESIAN_POINT ( 'NONE',  ( -4.999999999999998224, -44.99999999999997158, -99.00000000000000000 ) ) ;
#8634=MANIFOLD_SOLID_BREP ( 'Thread1', #1817 ) ;
#8637=ADVANCED_FACE ( 'NONE', ( #6738, #6080 ), #790, .F. ) ;
#8640=CARTESIAN_POINT ( 'NONE',  ( -3.535533905932736864, -41.46446609406723383, -99.90000000000000568 ) ) ;
#8642=CARTESIAN_POINT ( 'NONE',  ( 3.229347689422839895, -41.77065231057713390, -97.94999999890751496 ) ) ;
#8643=CARTESIAN_POINT ( 'NONE',  ( -1.377418269645616311, -49.84141567902239700, -99.99942299408148472 ) ) ;
#8646=CARTESIAN_POINT ( 'NONE',  ( 3.535533905932736420, -41.46446609406723383, -97.69300000002183992 ) ) ;
#8657=DIRECTION ( 'NONE',  ( -1.000000000000000000, 0.000000000000000000, -0.000000000000000000 ) ) ;
#8661=CARTESIAN_POINT ( 'NONE',  ( -3.229347689422839451, -48.22934768942280925, -99.34999999890752065 ) ) ;
#8672=CARTESIAN_POINT ( 'NONE',  ( 3.535533905932737309, -48.53553390593270933, -99.39999999781504414 ) ) ;
#8678=CARTESIAN_POINT ( 'NONE',  ( 4.566987299999998307, -43.10829192115428299, -98.99999999890751212 ) ) ;
#8679=CARTESIAN_POINT ( 'NONE',  ( -2.071067811865475505, -49.99999999999996447, -97.14999999781504414 ) ) ;
#8681=CARTESIAN_POINT ( 'NONE',  ( -4.566987299999998307, -44.99999999999997158, -96.84999999890753486 ) ) ;
#8682=CARTESIAN_POINT ( 'NONE',  ( -3.966436988140349396, -41.94266538335023142, -100.0008128833833894 ) ) ;
#8685=CARTESIAN_POINT ( 'NONE',  ( -4.999999999999997335, -47.07106781186546129, -96.54300000002183424 ) ) ;
#8700=CARTESIAN_POINT ( 'NONE',  ( 3.229347689422839895, -41.77065231057713390, -99.74999999890751212 ) ) ;
#8711=CARTESIAN_POINT ( 'NONE',  ( 4.999999999999998224, -44.99999999999997158, -97.69999999781505551 ) ) ;
#8712=CARTESIAN_POINT ( 'NONE',  ( 2.071067811865477282, -49.99999999999996447, -100.2499999978150669 ) ) ;
#8714=CARTESIAN_POINT ( 'NONE',  ( -4.999999999999998224, -44.99999999999997158, -98.19999999999998863 ) ) ;
#8716=EDGE_CURVE ( 'NONE', #6772, #7413, #1603, .T. ) ;
ENDSEC;
END-ISO-10303-21;
